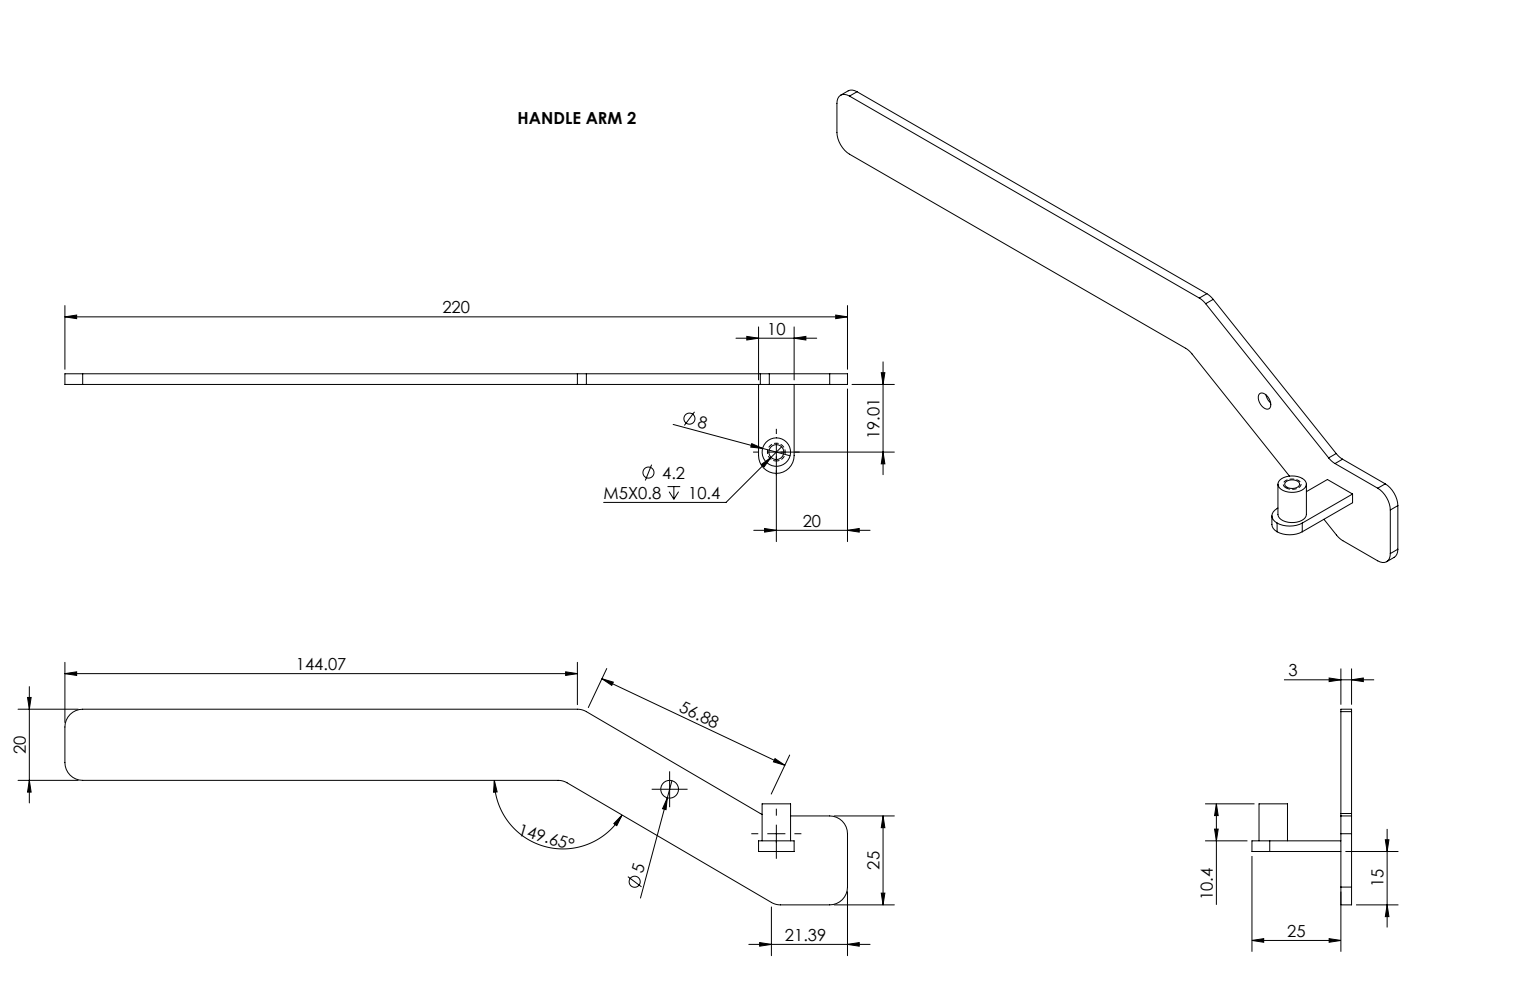
ISO-10303-21;
HEADER;
FILE_DESCRIPTION (('STEP AP214'),
    '1' );
FILE_NAME ('Handle arm 2.step',
    '2026-09-24T10:15:42',
    ( '' ),
    ( '' ),
    'SwSTEP 2.0',
    'SolidWorks 2026',
    '' );
FILE_SCHEMA (( 'AUTOMOTIVE_DESIGN' ));
ENDSEC;

DATA;
#2=DIRECTION ( 'NONE',  ( 0.000000000000000000, 0.000000000000000000, -1.000000000000000000 ) ) ;
#46=CARTESIAN_POINT ( 'NONE',  ( 3.686287386450715076E-15, -27.00000000000000000, 25.01316734529526187 ) ) ;
#85=EDGE_CURVE ( 'NONE', #9356, #911, #14003, .T. ) ;
#87=DIRECTION ( 'NONE',  ( 0.000000000000000000, 0.000000000000000000, 1.000000000000000000 ) ) ;
#167=AXIS2_PLACEMENT_3D ( 'NONE', #17284, #15857, #10023 ) ;
#171=CARTESIAN_POINT ( 'NONE',  ( 3.686287386450715076E-15, -16.60000000000000142, 27.11316734529526329 ) ) ;
#182=VERTEX_POINT ( 'NONE', #619 ) ;
#190=VECTOR ( 'NONE', #11538, 1000.000000000000000 ) ;
#196=DIRECTION ( 'NONE',  ( -0.000000000000000000, 1.000000000000000000, -0.000000000000000000 ) ) ;
#211=AXIS2_PLACEMENT_3D ( 'NONE', #14150, #17206, #1054 ) ;
#237=FACE_OUTER_BOUND ( 'NONE', #12508, .T. ) ;
#244=( LENGTH_UNIT ( ) NAMED_UNIT ( * ) SI_UNIT ( .MILLI., .METRE. ) );
#245=DIRECTION ( 'NONE',  ( 0.000000000000000000, 0.000000000000000000, 1.000000000000000000 ) ) ;
#255=ORIENTED_EDGE ( 'NONE', *, *, #85, .F. ) ;
#262=ORIENTED_EDGE ( 'NONE', *, *, #15287, .T. ) ;
#268=ADVANCED_FACE ( 'NONE', ( #16665 ), #15218, .F. ) ;
#282=EDGE_LOOP ( 'NONE', ( #350, #8843, #5301, #9575 ) ) ;
#335=CARTESIAN_POINT ( 'NONE',  ( -54.57590088527786065, 9.999999999999973355, 6.000000000000000000 ) ) ;
#350=ORIENTED_EDGE ( 'NONE', *, *, #847, .F. ) ;
#355=DIRECTION ( 'NONE',  ( -0.000000000000000000, 1.000000000000000000, -0.000000000000000000 ) ) ;
#372=DIRECTION ( 'NONE',  ( 0.000000000000000000, 0.000000000000000000, 1.000000000000000000 ) ) ;
#375=EDGE_CURVE ( 'NONE', #5396, #13349, #1164, .T. ) ;
#384=CARTESIAN_POINT ( 'NONE',  ( 20.00000000000000711, -45.00000000000000000, 6.000000000000000000 ) ) ;
#390=ORIENTED_EDGE ( 'NONE', *, *, #17273, .T. ) ;
#427=SURFACE_SIDE_STYLE ('',( #3278 ) ) ;
#479=PLANE ( 'NONE',  #15685 ) ;
#484=LINE ( 'NONE', #384, #10360 ) ;
#503=( GEOMETRIC_REPRESENTATION_CONTEXT ( 3 ) GLOBAL_UNCERTAINTY_ASSIGNED_CONTEXT ( ( #10335 ) ) GLOBAL_UNIT_ASSIGNED_CONTEXT ( ( #244, #6073, #17536 ) ) REPRESENTATION_CONTEXT ( 'NONE', 'WORKASPACE' ) );
#516=ORIENTED_EDGE ( 'NONE', *, *, #14577, .T. ) ;
#552=ORIENTED_EDGE ( 'NONE', *, *, #12638, .T. ) ;
#553=ORIENTED_EDGE ( 'NONE', *, *, #2654, .T. ) ;
#578=FACE_BOUND ( 'NONE', #591, .T. ) ;
#581=EDGE_CURVE ( 'NONE', #13464, #1391, #8679, .T. ) ;
#591=EDGE_LOOP ( 'NONE', ( #390, #2249 ) ) ;
#619=CARTESIAN_POINT ( 'NONE',  ( 15.00000000000000711, -45.00000000000000000, 6.000000000000000000 ) ) ;
#624=ADVANCED_FACE ( 'NONE', ( #14823 ), #6227, .F. ) ;
#647=CARTESIAN_POINT ( 'NONE',  ( 15.00000000000000711, -19.99999999999999645, 6.000000000000000000 ) ) ;
#656=ORIENTED_EDGE ( 'NONE', *, *, #2270, .T. ) ;
#720=CARTESIAN_POINT ( 'NONE',  ( -61.35602477868047799, -10.00000000000000888, 6.000000000000000000 ) ) ;
#722=EDGE_CURVE ( 'NONE', #14617, #1651, #2384, .T. ) ;
#738=VECTOR ( 'NONE', #4589, 1000.000000000000227 ) ;
#785=CARTESIAN_POINT ( 'NONE',  ( 5.000000000000006217, -30.00000000000000000, 6.000000000000000000 ) ) ;
#789=DIRECTION ( 'NONE',  ( 0.000000000000000000, 0.000000000000000000, -1.000000000000000000 ) ) ;
#825=CIRCLE ( 'NONE', #211, 5.000000000000004441 ) ;
#831=DIRECTION ( 'NONE',  ( 1.000000000000000000, 0.000000000000000000, 0.000000000000000000 ) ) ;
#836=CARTESIAN_POINT ( 'NONE',  ( 15.00000000000000711, -40.00000000000000000, 3.000000000000000000 ) ) ;
#840=ORIENTED_EDGE ( 'NONE', *, *, #14124, .T. ) ;
#846=VERTEX_POINT ( 'NONE', #13076 ) ;
#847=EDGE_CURVE ( 'NONE', #1377, #13406, #12495, .T. ) ;
#858=DIRECTION ( 'NONE',  ( -1.000000000000000000, -0.000000000000000000, -0.000000000000000000 ) ) ;
#904=CARTESIAN_POINT ( 'NONE',  ( 15.00000000000000711, -24.99999999999999645, 6.000000000000000000 ) ) ;
#911=VERTEX_POINT ( 'NONE', #7070 ) ;
#976=ADVANCED_FACE ( 'NONE', ( #6303 ), #14988, .F. ) ;
#983=CARTESIAN_POINT ( 'NONE',  ( -4.999999999999995559, -30.00000000000000000, 26.00000000000000000 ) ) ;
#994=ORIENTED_EDGE ( 'NONE', *, *, #17881, .T. ) ;
#998=VERTEX_POINT ( 'NONE', #13172 ) ;
#1009=AXIS2_PLACEMENT_3D ( 'NONE', #5627, #10227, #11663 ) ;
#1054=DIRECTION ( 'NONE',  ( -1.000000000000000000, 0.000000000000000000, 0.000000000000000000 ) ) ;
#1056=DIRECTION ( 'NONE',  ( 0.000000000000000000, 0.000000000000000000, -1.000000000000000000 ) ) ;
#1088=AXIS2_PLACEMENT_3D ( 'NONE', #17339, #4255, #4345 ) ;
#1150=LINE ( 'NONE', #9834, #4116 ) ;
#1156=FACE_OUTER_BOUND ( 'NONE', #9724, .T. ) ;
#1164=CIRCLE ( 'NONE', #7602, 5.000000000000004441 ) ;
#1180=DIRECTION ( 'NONE',  ( 0.000000000000000000, 0.000000000000000000, 1.000000000000000000 ) ) ;
#1181=DIRECTION ( 'NONE',  ( -0.000000000000000000, -0.000000000000000000, -1.000000000000000000 ) ) ;
#1190=ORIENTED_EDGE ( 'NONE', *, *, #7855, .T. ) ;
#1216=CARTESIAN_POINT ( 'NONE',  ( -4.505465888036630062, -19.31487138727242581, 6.000000000000000000 ) ) ;
#1227=DIRECTION ( 'NONE',  ( 0.000000000000000000, 0.000000000000000000, -1.000000000000000000 ) ) ;
#1238=DIRECTION ( 'NONE',  ( -0.000000000000000000, -0.000000000000000000, 1.000000000000000000 ) ) ;
#1254=CARTESIAN_POINT ( 'NONE',  ( 20.00000000000000711, -24.99999999999999645, 6.000000000000000000 ) ) ;
#1255=FACE_OUTER_BOUND ( 'NONE', #3235, .T. ) ;
#1285=EDGE_CURVE ( 'NONE', #10015, #2548, #5780, .T. ) ;
#1289=LINE ( 'NONE', #9710, #13681 ) ;
#1297=ORIENTED_EDGE ( 'NONE', *, *, #5077, .T. ) ;
#1326=CARTESIAN_POINT ( 'NONE',  ( -54.57590088527786065, 9.999999999999973355, 6.000000000000000000 ) ) ;
#1336=FACE_OUTER_BOUND ( 'NONE', #12011, .T. ) ;
#1377=VERTEX_POINT ( 'NONE', #7431 ) ;
#1391=VERTEX_POINT ( 'NONE', #12012 ) ;
#1419=CARTESIAN_POINT ( 'NONE',  ( 4.336808689942014581E-15, -27.00000000000000000, 26.00000000000000000 ) ) ;
#1431=AXIS2_PLACEMENT_3D ( 'NONE', #13888, #9216, #7903 ) ;
#1441=FACE_OUTER_BOUND ( 'NONE', #12105, .T. ) ;
#1454=DIRECTION ( 'NONE',  ( -0.000000000000000000, -0.000000000000000000, -1.000000000000000000 ) ) ;
#1517=ORIENTED_EDGE ( 'NONE', *, *, #11103, .F. ) ;
#1518=VERTEX_POINT ( 'NONE', #13981 ) ;
#1519=ORIENTED_EDGE ( 'NONE', *, *, #5489, .T. ) ;
#1529=DIRECTION ( 'NONE',  ( -0.000000000000000000, 1.000000000000000000, -0.000000000000000000 ) ) ;
#1546=DIRECTION ( 'NONE',  ( -0.000000000000000000, -0.000000000000000000, 1.000000000000000000 ) ) ;
#1578=LINE ( 'NONE', #7419, #10628 ) ;
#1586=EDGE_CURVE ( 'NONE', #1391, #14370, #11676, .T. ) ;
#1590=ORIENTED_EDGE ( 'NONE', *, *, #9778, .T. ) ;
#1591=LINE ( 'NONE', #7435, #8998 ) ;
#1605=EDGE_LOOP ( 'NONE', ( #14578, #7944, #5603, #3741, #6106 ) ) ;
#1651=VERTEX_POINT ( 'NONE', #10339 ) ;
#1708=DIRECTION ( 'NONE',  ( 0.000000000000000000, -1.000000000000000000, 0.000000000000000000 ) ) ;
#1717=PLANE ( 'NONE',  #10053 ) ;
#1735=DIRECTION ( 'NONE',  ( -0.8629742774544859607, 0.5052478564545405115, 0.000000000000000000 ) ) ;
#1738=ORIENTED_EDGE ( 'NONE', *, *, #18088, .F. ) ;
#1764=FILL_AREA_STYLE ('',( #3572 ) ) ;
#1774=DIRECTION ( 'NONE',  ( -0.000000000000000000, -0.000000000000000000, 1.000000000000000000 ) ) ;
#1809=DIRECTION ( 'NONE',  ( 0.000000000000000000, 1.000000000000000000, -0.000000000000000000 ) ) ;
#1813=CARTESIAN_POINT ( 'NONE',  ( -53.40568638168567617, 9.314871387272408043, 6.000000000000000000 ) ) ;
#1816=EDGE_CURVE ( 'NONE', #15520, #5678, #15774, .T. ) ;
#1868=DIRECTION ( 'NONE',  ( -1.000000000000000000, -1.387778780781445676E-15, 0.000000000000000000 ) ) ;
#1869=ADVANCED_FACE ( 'NONE', ( #12519 ), #10124, .F. ) ;
#1871=CARTESIAN_POINT ( 'NONE',  ( -58.82978549640777288, -10.68512861272757952, 6.000000000000000000 ) ) ;
#1882=EDGE_LOOP ( 'NONE', ( #10890, #7353 ) ) ;
#1890=ADVANCED_FACE ( 'NONE', ( #10319 ), #15948, .T. ) ;
#1897=DIRECTION ( 'NONE',  ( 0.000000000000000000, -1.000000000000000000, 0.000000000000000000 ) ) ;
#1903=ORIENTED_EDGE ( 'NONE', *, *, #8948, .T. ) ;
#1915=CARTESIAN_POINT ( 'NONE',  ( 3.686287386450715076E-15, -16.60000000000000142, 27.11316734529526329 ) ) ;
#1919=EDGE_CURVE ( 'NONE', #7625, #1518, #14240, .T. ) ;
#1942=EDGE_LOOP ( 'NONE', ( #12597, #3775, #16274, #14695 ) ) ;
#1963=PLANE ( 'NONE',  #5380 ) ;
#1978=ORIENTED_EDGE ( 'NONE', *, *, #8575, .T. ) ;
#1985=DIRECTION ( 'NONE',  ( 1.000000000000000000, 0.000000000000000000, 0.000000000000000000 ) ) ;
#2030=AXIS2_PLACEMENT_3D ( 'NONE', #15716, #11248, #17249 ) ;
#2054=VECTOR ( 'NONE', #11619, 1000.000000000000000 ) ;
#2059=DIRECTION ( 'NONE',  ( 0.000000000000000000, 0.000000000000000000, -1.000000000000000000 ) ) ;
#2077=EDGE_LOOP ( 'NONE', ( #13785, #14387, #12473, #3682 ) ) ;
#2078=ORIENTED_EDGE ( 'NONE', *, *, #17877, .T. ) ;
#2199=LINE ( 'NONE', #16475, #8487 ) ;
#2216=LINE ( 'NONE', #785, #17824 ) ;
#2244=EDGE_CURVE ( 'NONE', #18846, #1377, #4850, .T. ) ;
#2249=ORIENTED_EDGE ( 'NONE', *, *, #2491, .T. ) ;
#2262=DIRECTION ( 'NONE',  ( -0.000000000000000000, -0.000000000000000000, -1.000000000000000000 ) ) ;
#2270=EDGE_CURVE ( 'NONE', #9430, #14370, #1591, .T. ) ;
#2274=ORIENTED_EDGE ( 'NONE', *, *, #18088, .T. ) ;
#2280=CARTESIAN_POINT ( 'NONE',  ( -55.93192566395838128, 9.999999999999973355, 6.000000000000000000 ) ) ;
#2298=CYLINDRICAL_SURFACE ( 'NONE', #3949, 2.499999999999992006 ) ;
#2316=VERTEX_POINT ( 'NONE', #16125 ) ;
#2335=CARTESIAN_POINT ( 'NONE',  ( -30.00000000000000355, -12.50000000000000178, 3.000000000000000000 ) ) ;
#2356=DIRECTION ( 'NONE',  ( -1.000000000000000000, 0.000000000000000000, 0.000000000000000000 ) ) ;
#2371=AXIS2_PLACEMENT_3D ( 'NONE', #17344, #17739, #11904 ) ;
#2382=EDGE_CURVE ( 'NONE', #13257, #7625, #18395, .T. ) ;
#2384=LINE ( 'NONE', #15566, #10687 ) ;
#2394=CARTESIAN_POINT ( 'NONE',  ( -61.35602477868047799, -15.00000000000000711, 6.000000000000000000 ) ) ;
#2491=EDGE_CURVE ( 'NONE', #2548, #14769, #13939, .T. ) ;
#2504=DIRECTION ( 'NONE',  ( -1.000000000000000000, 0.000000000000000000, 0.000000000000000000 ) ) ;
#2511=ORIENTED_EDGE ( 'NONE', *, *, #3757, .T. ) ;
#2528=EDGE_CURVE ( 'NONE', #7625, #15007, #18216, .T. ) ;
#2541=PRODUCT_DEFINITION_FORMATION_WITH_SPECIFIED_SOURCE ( 'ANY', '', #12278, .NOT_KNOWN. ) ;
#2548=VERTEX_POINT ( 'NONE', #5961 ) ;
#2566=EDGE_CURVE ( 'NONE', #18408, #6600, #3875, .T. ) ;
#2588=DIRECTION ( 'NONE',  ( 1.000000000000000000, -0.000000000000000000, -0.000000000000000000 ) ) ;
#2595=CARTESIAN_POINT ( 'NONE',  ( -59.99999999999997158, -10.00000000000000888, 6.000000000000000000 ) ) ;
#2605=ORIENTED_EDGE ( 'NONE', *, *, #2244, .T. ) ;
#2647=AXIS2_PLACEMENT_3D ( 'NONE', #6461, #6559, #18480 ) ;
#2649=ORIENTED_EDGE ( 'NONE', *, *, #9078, .F. ) ;
#2652=ORIENTED_EDGE ( 'NONE', *, *, #14147, .F. ) ;
#2654=EDGE_CURVE ( 'NONE', #15726, #12603, #6937, .T. ) ;
#2689=CARTESIAN_POINT ( 'NONE',  ( -30.00000000000000355, -12.50000000000000178, 6.000000000000000000 ) ) ;
#2695=EDGE_CURVE ( 'NONE', #9382, #15782, #9499, .T. ) ;
#2709=( NAMED_UNIT ( * ) SI_UNIT ( $, .STERADIAN. ) SOLID_ANGLE_UNIT ( ) );
#2724=ORIENTED_EDGE ( 'NONE', *, *, #4872, .F. ) ;
#2744=LINE ( 'NONE', #1326, #5606 ) ;
#2770=DIRECTION ( 'NONE',  ( -1.000000000000000000, 0.000000000000000000, 0.000000000000000000 ) ) ;
#2803=VERTEX_POINT ( 'NONE', #983 ) ;
#2805=VERTEX_POINT ( 'NONE', #8433 ) ;
#2830=VECTOR ( 'NONE', #196, 1000.000000000000000 ) ;
#2892=AXIS2_PLACEMENT_3D ( 'NONE', #15262, #831, #14097 ) ;
#2895=CARTESIAN_POINT ( 'NONE',  ( -53.40568638168567617, 9.314871387272408043, 3.000000000000000000 ) ) ;
#2902=AXIS2_PLACEMENT_3D ( 'NONE', #12160, #10430, #8893 ) ;
#2918=VECTOR ( 'NONE', #16196, 1000.000000000000000 ) ;
#2931=ORIENTED_EDGE ( 'NONE', *, *, #722, .T. ) ;
#2939=AXIS2_PLACEMENT_3D ( 'NONE', #7030, #12844, #11425 ) ;
#2988=CARTESIAN_POINT ( 'NONE',  ( 3.686287386450715076E-15, -27.00000000000000000, 25.01316734529526187 ) ) ;
#2990=DIRECTION ( 'NONE',  ( 0.000000000000000000, 0.000000000000000000, -1.000000000000000000 ) ) ;
#3016=AXIS2_PLACEMENT_3D ( 'NONE', #6543, #17924, #13612 ) ;
#3048=CARTESIAN_POINT ( 'NONE',  ( -0.2192422490275049152, -45.00000000000000000, 6.000000000000000000 ) ) ;
#3049=UNCERTAINTY_MEASURE_WITH_UNIT (LENGTH_MEASURE( 1.000000000000000082E-05 ), #15530, 'distance_accuracy_value', 'NONE');
#3053=CARTESIAN_POINT ( 'NONE',  ( 15.00000000000000711, -24.99999999999999645, 6.000000000000000000 ) ) ;
#3055=CARTESIAN_POINT ( 'NONE',  ( 20.00000000000000711, -40.00000000000000000, 6.000000000000000000 ) ) ;
#3089=PRODUCT_DEFINITION ( 'UNKNOWN', '', #2541, #4217 ) ;
#3113=ORIENTED_EDGE ( 'NONE', *, *, #14292, .T. ) ;
#3126=CARTESIAN_POINT ( 'NONE',  ( -4.999999999999995559, -27.00000000000000000, 31.00000000000000000 ) ) ;
#3143=VECTOR ( 'NONE', #17164, 1000.000000000000000 ) ;
#3145=VERTEX_POINT ( 'NONE', #14221 ) ;
#3169=VERTEX_POINT ( 'NONE', #9908 ) ;
#3179=LINE ( 'NONE', #4545, #8102 ) ;
#3182=CARTESIAN_POINT ( 'NONE',  ( -194.9999999999999716, -5.000000000000024869, 3.000000000000000000 ) ) ;
#3187=AXIS2_PLACEMENT_3D ( 'NONE', #18811, #1708, #7167 ) ;
#3225=DIRECTION ( 'NONE',  ( 0.000000000000000000, -1.000000000000000000, 0.000000000000000000 ) ) ;
#3235=EDGE_LOOP ( 'NONE', ( #3338, #5545, #6726, #16756 ) ) ;
#3246=ORIENTED_EDGE ( 'NONE', *, *, #2566, .T. ) ;
#3251=ORIENTED_EDGE ( 'NONE', *, *, #8948, .F. ) ;
#3258=CIRCLE ( 'NONE', #13950, 5.000000000000000888 ) ;
#3260=ORIENTED_EDGE ( 'NONE', *, *, #13945, .T. ) ;
#3265=FACE_OUTER_BOUND ( 'NONE', #14790, .T. ) ;
#3271=EDGE_CURVE ( 'NONE', #12603, #4207, #17956, .T. ) ;
#3278=SURFACE_STYLE_FILL_AREA ( #1764 ) ;
#3283=FILL_AREA_STYLE ('',( #14663 ) ) ;
#3291=EDGE_LOOP ( 'NONE', ( #11241, #8275, #18451, #8539 ) ) ;
#3310=CARTESIAN_POINT ( 'NONE',  ( 3.686287386450715076E-15, -16.60000000000000142, 25.01316734529526187 ) ) ;
#3338=ORIENTED_EDGE ( 'NONE', *, *, #15287, .F. ) ;
#3364=DIRECTION ( 'NONE',  ( -1.000000000000000000, 0.000000000000000000, 0.000000000000000000 ) ) ;
#3379=CARTESIAN_POINT ( 'NONE',  ( 4.336808689942017736E-15, 0.000000000000000000, 31.00000000000000000 ) ) ;
#3402=VECTOR ( 'NONE', #3460, 1000.000000000000000 ) ;
#3414=AXIS2_PLACEMENT_3D ( 'NONE', #16438, #372, #16716 ) ;
#3444=CIRCLE ( 'NONE', #7737, 5.000000000000004441 ) ;
#3445=ORIENTED_EDGE ( 'NONE', *, *, #11834, .F. ) ;
#3457=LINE ( 'NONE', #13493, #16294 ) ;
#3460=DIRECTION ( 'NONE',  ( -0.8629742774544855166, 0.5052478564545411777, -0.000000000000000000 ) ) ;
#3480=DIRECTION ( 'NONE',  ( 5.782411586589358625E-16, -1.000000000000000000, -0.000000000000000000 ) ) ;
#3493=ORIENTED_EDGE ( 'NONE', *, *, #11591, .F. ) ;
#3521=ADVANCED_FACE ( 'NONE', ( #237 ), #11349, .T. ) ;
#3553=MANIFOLD_SOLID_BREP ( 'AdvancedHole1', #9975 ) ;
#3563=VERTEX_POINT ( 'NONE', #6162 ) ;
#3565=DIRECTION ( 'NONE',  ( 0.000000000000000000, 0.000000000000000000, 1.000000000000000000 ) ) ;
#3572=FILL_AREA_STYLE_COLOUR ( '', #16481 ) ;
#3603=EDGE_CURVE ( 'NONE', #10015, #2805, #7629, .T. ) ;
#3604=PLANE ( 'NONE',  #2892 ) ;
#3671=PRODUCT_CONTEXT ( 'NONE', #11932, 'mechanical' ) ;
#3675=CIRCLE ( 'NONE', #4289, 4.000000000000000000 ) ;
#3682=ORIENTED_EDGE ( 'NONE', *, *, #16814, .F. ) ;
#3695=ADVANCED_FACE ( 'NONE', ( #6642 ), #7005, .T. ) ;
#3696=LINE ( 'NONE', #15350, #10169 ) ;
#3741=ORIENTED_EDGE ( 'NONE', *, *, #4041, .T. ) ;
#3755=ADVANCED_FACE ( 'NONE', ( #1255 ), #15970, .T. ) ;
#3757=EDGE_CURVE ( 'NONE', #2803, #14617, #12914, .T. ) ;
#3775=ORIENTED_EDGE ( 'NONE', *, *, #18129, .T. ) ;
#3782=FACE_OUTER_BOUND ( 'NONE', #6562, .T. ) ;
#3815=AXIS2_PLACEMENT_3D ( 'NONE', #4441, #8744, #14567 ) ;
#3817=EDGE_LOOP ( 'NONE', ( #9700, #10501, #8493, #2511, #2931 ) ) ;
#3828=CARTESIAN_POINT ( 'NONE',  ( -4.999999999999995559, -27.00000000000000000, 6.000000000000000000 ) ) ;
#3841=AXIS2_PLACEMENT_3D ( 'NONE', #17972, #12233, #16622 ) ;
#3875=CIRCLE ( 'NONE', #9061, 5.000000000000000000 ) ;
#3881=AXIS2_PLACEMENT_3D ( 'NONE', #8923, #13711, #7705 ) ;
#3898=CARTESIAN_POINT ( 'NONE',  ( 5.000000000000004441, -27.00000000000000000, 31.00000000000000000 ) ) ;
#3906=CIRCLE ( 'NONE', #17034, 5.000000000000000000 ) ;
#3912=FACE_OUTER_BOUND ( 'NONE', #7626, .T. ) ;
#3915=ADVANCED_FACE ( 'NONE', ( #18266 ), #2298, .F. ) ;
#3935=CARTESIAN_POINT ( 'NONE',  ( -199.9999999999999716, -10.00000000000002665, 6.000000000000000000 ) ) ;
#3949=AXIS2_PLACEMENT_3D ( 'NONE', #5355, #15392, #10924 ) ;
#3958=DIRECTION ( 'NONE',  ( 1.000000000000000000, 0.000000000000000000, 0.000000000000000000 ) ) ;
#3959=DIRECTION ( 'NONE',  ( -0.000000000000000000, -1.000000000000000000, -0.000000000000000000 ) ) ;
#3962=VERTEX_POINT ( 'NONE', #3828 ) ;
#3980=ORIENTED_EDGE ( 'NONE', *, *, #8436, .F. ) ;
#3986=ORIENTED_EDGE ( 'NONE', *, *, #15577, .T. ) ;
#3995=FACE_OUTER_BOUND ( 'NONE', #9987, .T. ) ;
#4022=CARTESIAN_POINT ( 'NONE',  ( -199.9999999999999716, -5.000000000000024869, 6.000000000000000000 ) ) ;
#4041=EDGE_CURVE ( 'NONE', #3145, #3962, #14334, .T. ) ;
#4059=CIRCLE ( 'NONE', #11680, 4.000000000000000000 ) ;
#4113=AXIS2_PLACEMENT_3D ( 'NONE', #17385, #10217, #11564 ) ;
#4116=VECTOR ( 'NONE', #16051, 1000.000000000000227 ) ;
#4135=EDGE_CURVE ( 'NONE', #12673, #911, #18818, .T. ) ;
#4158=MECHANICAL_DESIGN_GEOMETRIC_PRESENTATION_REPRESENTATION('',(#6598),#503);
#4175=ORIENTED_EDGE ( 'NONE', *, *, #4872, .T. ) ;
#4207=VERTEX_POINT ( 'NONE', #1915 ) ;
#4211=CARTESIAN_POINT ( 'NONE',  ( 3.686287386450715076E-15, -27.00000000000000000, 25.01316734529526187 ) ) ;
#4217=PRODUCT_DEFINITION_CONTEXT ( 'detailed design', #14375, 'design' ) ;
#4255=DIRECTION ( 'NONE',  ( -0.000000000000000000, -0.000000000000000000, 1.000000000000000000 ) ) ;
#4264=AXIS2_PLACEMENT_3D ( 'NONE', #8501, #1227, #7165 ) ;
#4272=CARTESIAN_POINT ( 'NONE',  ( 4.176146106109656457E-15, -16.60000000000000142, 29.01316734529526187 ) ) ;
#4289=AXIS2_PLACEMENT_3D ( 'NONE', #4211, #5813, #9832 ) ;
#4306=LINE ( 'NONE', #5817, #2830 ) ;
#4322=DIRECTION ( 'NONE',  ( -1.000000000000000000, 0.000000000000000000, 0.000000000000000000 ) ) ;
#4345=DIRECTION ( 'NONE',  ( -1.000000000000000000, 0.000000000000000000, 0.000000000000000000 ) ) ;
#4350=SURFACE_STYLE_FILL_AREA ( #3283 ) ;
#4377=ORIENTED_EDGE ( 'NONE', *, *, #5439, .T. ) ;
#4384=AXIS2_PLACEMENT_3D ( 'NONE', #9240, #4564, #1985 ) ;
#4408=AXIS2_PLACEMENT_3D ( 'NONE', #12984, #11657, #8506 ) ;
#4413=EDGE_CURVE ( 'NONE', #3962, #14617, #15736, .T. ) ;
#4431=ORIENTED_EDGE ( 'NONE', *, *, #16809, .T. ) ;
#4441=CARTESIAN_POINT ( 'NONE',  ( -4.999999999999995559, -30.00000000000000000, 31.00000000000000000 ) ) ;
#4444=PRESENTATION_STYLE_ASSIGNMENT (( #7417 ) ) ;
#4453=ORIENTED_EDGE ( 'NONE', *, *, #2566, .F. ) ;
#4454=EDGE_LOOP ( 'NONE', ( #8547, #16780, #7578 ) ) ;
#4456=CIRCLE ( 'NONE', #1088, 5.000000000000004441 ) ;
#4498=CARTESIAN_POINT ( 'NONE',  ( -199.9999999999999716, -10.00000000000002665, 6.000000000000000000 ) ) ;
#4545=CARTESIAN_POINT ( 'NONE',  ( -59.99999999999997158, -10.00000000000000888, 3.000000000000000000 ) ) ;
#4548=FACE_OUTER_BOUND ( 'NONE', #7524, .T. ) ;
#4561=DIRECTION ( 'NONE',  ( -1.000000000000000000, -5.782411586589358625E-16, 0.000000000000000000 ) ) ;
#4564=DIRECTION ( 'NONE',  ( 0.000000000000000000, 0.000000000000000000, 1.000000000000000000 ) ) ;
#4570=DIRECTION ( 'NONE',  ( 0.000000000000000000, 0.000000000000000000, -1.000000000000000000 ) ) ;
#4577=ORIENTED_EDGE ( 'NONE', *, *, #12513, .T. ) ;
#4584=CARTESIAN_POINT ( 'NONE',  ( -55.93192566395838128, 9.999999999999973355, 3.000000000000000000 ) ) ;
#4589=DIRECTION ( 'NONE',  ( 0.8629742774544859607, -0.5052478564545405115, -0.000000000000000000 ) ) ;
#4590=DIRECTION ( 'NONE',  ( 1.000000000000000000, 0.000000000000000000, 0.000000000000000000 ) ) ;
#4627=CARTESIAN_POINT ( 'NONE',  ( 3.686287386450715076E-15, -27.00000000000000000, 25.01316734529526187 ) ) ;
#4643=CARTESIAN_POINT ( 'NONE',  ( -199.9999999999999716, -5.000000000000024869, 6.000000000000000000 ) ) ;
#4644=EDGE_CURVE ( 'NONE', #14303, #15038, #13554, .T. ) ;
#4648=ORIENTED_EDGE ( 'NONE', *, *, #2382, .F. ) ;
#4684=DIRECTION ( 'NONE',  ( 0.000000000000000000, 0.000000000000000000, 1.000000000000000000 ) ) ;
#4706=DIRECTION ( 'NONE',  ( 1.049727191138619928E-16, 0.5150380749100523792, -0.8571673007021134438 ) ) ;
#4736=DIRECTION ( 'NONE',  ( -1.000000000000000000, 0.000000000000000000, 0.000000000000000000 ) ) ;
#4758=DIRECTION ( 'NONE',  ( -0.000000000000000000, 1.000000000000000000, -0.000000000000000000 ) ) ;
#4769=EDGE_CURVE ( 'NONE', #846, #3169, #11560, .T. ) ;
#4789=LINE ( 'NONE', #12247, #16996 ) ;
#4840=LINE ( 'NONE', #720, #11810 ) ;
#4850=LINE ( 'NONE', #7633, #18753 ) ;
#4872=EDGE_CURVE ( 'NONE', #13406, #8344, #2744, .T. ) ;
#4882=( GEOMETRIC_REPRESENTATION_CONTEXT ( 3 ) GLOBAL_UNCERTAINTY_ASSIGNED_CONTEXT ( ( #11314 ) ) GLOBAL_UNIT_ASSIGNED_CONTEXT ( ( #10749, #6361, #15236 ) ) REPRESENTATION_CONTEXT ( 'NONE', 'WORKASPACE' ) );
#4920=PRESENTATION_STYLE_ASSIGNMENT (( #15043 ) ) ;
#4929=CARTESIAN_POINT ( 'NONE',  ( -27.50000000000000711, -12.50000000000000178, 3.000000000000000000 ) ) ;
#4957=ADVANCED_FACE ( 'NONE', ( #7748, #13370 ), #479, .F. ) ;
#4963=PLANE ( 'NONE',  #5345 ) ;
#4992=ORIENTED_EDGE ( 'NONE', *, *, #1919, .T. ) ;
#5010=ADVANCED_FACE ( 'NONE', ( #5475 ), #5744, .F. ) ;
#5077=EDGE_CURVE ( 'NONE', #18014, #2316, #16619, .T. ) ;
#5082=CARTESIAN_POINT ( 'NONE',  ( -54.57590088527786065, 9.999999999999973355, 3.000000000000000000 ) ) ;
#5098=VECTOR ( 'NONE', #1181, 1000.000000000000000 ) ;
#5106=VECTOR ( 'NONE', #1546, 1000.000000000000000 ) ;
#5115=CARTESIAN_POINT ( 'NONE',  ( 3.943463214271659518E-15, -16.60000000000000142, 22.91316734529526045 ) ) ;
#5130=CARTESIAN_POINT ( 'NONE',  ( 15.00000000000000711, -40.00000000000000000, 6.000000000000000000 ) ) ;
#5145=LINE ( 'NONE', #3898, #14518 ) ;
#5176=CARTESIAN_POINT ( 'NONE',  ( 15.00000000000000711, -19.99999999999999645, 6.000000000000000000 ) ) ;
#5212=ORIENTED_EDGE ( 'NONE', *, *, #14729, .T. ) ;
#5225=CARTESIAN_POINT ( 'NONE',  ( -1.389456752619696367, -44.31487138727242581, 6.000000000000000000 ) ) ;
#5301=ORIENTED_EDGE ( 'NONE', *, *, #14124, .F. ) ;
#5319=VECTOR ( 'NONE', #16971, 1000.000000000000000 ) ;
#5327=ORIENTED_EDGE ( 'NONE', *, *, #17881, .F. ) ;
#5335=PLANE ( 'NONE',  #7776 ) ;
#5345=AXIS2_PLACEMENT_3D ( 'NONE', #3126, #3225, #7943 ) ;
#5347=EDGE_CURVE ( 'NONE', #3169, #1518, #825, .T. ) ;
#5355=CARTESIAN_POINT ( 'NONE',  ( -30.00000000000000355, -12.50000000000000178, 6.000000000000000000 ) ) ;
#5360=CARTESIAN_POINT ( 'NONE',  ( -32.49999999999999289, -12.50000000000000178, 6.000000000000000000 ) ) ;
#5380=AXIS2_PLACEMENT_3D ( 'NONE', #335, #13226, #6163 ) ;
#5396=VERTEX_POINT ( 'NONE', #4022 ) ;
#5398=ORIENTED_EDGE ( 'NONE', *, *, #4135, .T. ) ;
#5406=DIRECTION ( 'NONE',  ( 0.000000000000000000, 0.000000000000000000, -1.000000000000000000 ) ) ;
#5439=EDGE_CURVE ( 'NONE', #5705, #10186, #7549, .T. ) ;
#5462=DIRECTION ( 'NONE',  ( 0.000000000000000000, -1.000000000000000000, 0.000000000000000000 ) ) ;
#5463=CIRCLE ( 'NONE', #6402, 2.100000000000000977 ) ;
#5475=FACE_OUTER_BOUND ( 'NONE', #13295, .T. ) ;
#5478=ORIENTED_EDGE ( 'NONE', *, *, #1586, .T. ) ;
#5481=ORIENTED_EDGE ( 'NONE', *, *, #13945, .F. ) ;
#5489=EDGE_CURVE ( 'NONE', #12673, #16909, #6319, .T. ) ;
#5535=CARTESIAN_POINT ( 'NONE',  ( 3.686287386450715076E-15, -27.00000000000000000, 27.11316734529526329 ) ) ;
#5541=EDGE_LOOP ( 'NONE', ( #1297, #12434, #16868, #17434 ) ) ;
#5545=ORIENTED_EDGE ( 'NONE', *, *, #1586, .F. ) ;
#5556=CARTESIAN_POINT ( 'NONE',  ( -30.00000000000000355, -12.50000000000000178, 6.000000000000000000 ) ) ;
#5600=CARTESIAN_POINT ( 'NONE',  ( -194.9999999999999716, -10.00000000000002665, 6.000000000000000000 ) ) ;
#5603=ORIENTED_EDGE ( 'NONE', *, *, #8436, .T. ) ;
#5606=VECTOR ( 'NONE', #18812, 1000.000000000000000 ) ;
#5627=CARTESIAN_POINT ( 'NONE',  ( 3.686287386450715076E-15, -16.60000000000000142, 25.01316734529526187 ) ) ;
#5647=CONICAL_SURFACE ( 'NONE', #12674, 2.100000000000000977, 1.029744258676656532 ) ;
#5661=ORIENTED_EDGE ( 'NONE', *, *, #9078, .T. ) ;
#5678=VERTEX_POINT ( 'NONE', #15290 ) ;
#5705=VERTEX_POINT ( 'NONE', #17546 ) ;
#5724=ADVANCED_FACE ( 'NONE', ( #8495 ), #14322, .T. ) ;
#5731=ORIENTED_EDGE ( 'NONE', *, *, #14910, .F. ) ;
#5734=ADVANCED_FACE ( 'NONE', ( #3912 ), #15471, .F. ) ;
#5744=CYLINDRICAL_SURFACE ( 'NONE', #9288, 4.999999999999997335 ) ;
#5759=VECTOR ( 'NONE', #14419, 1000.000000000000000 ) ;
#5780=LINE ( 'NONE', #4272, #3143 ) ;
#5797=SHAPE_REPRESENTATION ( 'Handle arm 2', ( #2030 ), #14825 ) ;
#5813=DIRECTION ( 'NONE',  ( 0.000000000000000000, -1.000000000000000000, 0.000000000000000000 ) ) ;
#5817=CARTESIAN_POINT ( 'NONE',  ( 20.00000000000000711, -19.99999999999999645, 3.000000000000000000 ) ) ;
#5822=DIRECTION ( 'NONE',  ( -0.000000000000000000, -0.000000000000000000, 1.000000000000000000 ) ) ;
#5863=PLANE ( 'NONE',  #3815 ) ;
#5870=EDGE_LOOP ( 'NONE', ( #15390, #7937 ) ) ;
#5871=CARTESIAN_POINT ( 'NONE',  ( 3.686287386450715076E-15, -16.60000000000000142, 25.01316734529526187 ) ) ;
#5873=CIRCLE ( 'NONE', #14732, 2.100000000000000977 ) ;
#5890=CYLINDRICAL_SURFACE ( 'NONE', #17248, 4.000000000000000000 ) ;
#5898=VERTEX_POINT ( 'NONE', #5115 ) ;
#5911=FACE_OUTER_BOUND ( 'NONE', #8521, .T. ) ;
#5924=ADVANCED_FACE ( 'NONE', ( #16960 ), #9594, .F. ) ;
#5934=CARTESIAN_POINT ( 'NONE',  ( 3.943463214271659518E-15, -27.00000000000000000, 22.91316734529526045 ) ) ;
#5957=DIRECTION ( 'NONE',  ( 0.000000000000000000, 0.000000000000000000, -1.000000000000000000 ) ) ;
#5961=CARTESIAN_POINT ( 'NONE',  ( 4.176146106109656457E-15, -27.00000000000000000, 29.01316734529526187 ) ) ;
#6028=DIRECTION ( 'NONE',  ( -1.000000000000000000, 0.000000000000000000, 0.000000000000000000 ) ) ;
#6062=ORIENTED_EDGE ( 'NONE', *, *, #14577, .F. ) ;
#6073=( NAMED_UNIT ( * ) PLANE_ANGLE_UNIT ( ) SI_UNIT ( $, .RADIAN. ) );
#6080=VECTOR ( 'NONE', #5462, 1000.000000000000000 ) ;
#6106=ORIENTED_EDGE ( 'NONE', *, *, #15840, .F. ) ;
#6114=DIRECTION ( 'NONE',  ( 0.000000000000000000, -1.000000000000000000, 0.000000000000000000 ) ) ;
#6162=CARTESIAN_POINT ( 'NONE',  ( 4.336808689942017736E-15, -30.00000000000000000, 31.00000000000000000 ) ) ;
#6163=DIRECTION ( 'NONE',  ( 0.8629742774544855166, -0.5052478564545411777, 0.000000000000000000 ) ) ;
#6166=CARTESIAN_POINT ( 'NONE',  ( -58.82978549640777288, -10.68512861272758308, 3.000000000000000000 ) ) ;
#6168=DIRECTION ( 'NONE',  ( -1.000000000000000000, 0.000000000000000000, 0.000000000000000000 ) ) ;
#6171=LINE ( 'NONE', #4643, #2054 ) ;
#6227=PLANE ( 'NONE',  #18489 ) ;
#6243=ORIENTED_EDGE ( 'NONE', *, *, #15577, .F. ) ;
#6303=FACE_OUTER_BOUND ( 'NONE', #7291, .T. ) ;
#6318=ORIENTED_EDGE ( 'NONE', *, *, #7855, .F. ) ;
#6319=CIRCLE ( 'NONE', #16987, 5.000000000000004441 ) ;
#6323=DIRECTION ( 'NONE',  ( -0.000000000000000000, -0.000000000000000000, -1.000000000000000000 ) ) ;
#6324=VECTOR ( 'NONE', #15842, 1000.000000000000000 ) ;
#6331=PRODUCT_DEFINITION_SHAPE ( 'NONE', 'NONE',  #3089 ) ;
#6337=LINE ( 'NONE', #5934, #16471 ) ;
#6361=( NAMED_UNIT ( * ) PLANE_ANGLE_UNIT ( ) SI_UNIT ( $, .RADIAN. ) );
#6364=CARTESIAN_POINT ( 'NONE',  ( 5.000000000000006217, -30.00000000000000000, 26.00000000000000000 ) ) ;
#6402=AXIS2_PLACEMENT_3D ( 'NONE', #14613, #1529, #4684 ) ;
#6461=CARTESIAN_POINT ( 'NONE',  ( -59.99999999999997158, -10.00000000000000888, 6.000000000000000000 ) ) ;
#6523=CARTESIAN_POINT ( 'NONE',  ( 3.686287386450715076E-15, -28.26180729995786933, 25.01316734529526187 ) ) ;
#6543=CARTESIAN_POINT ( 'NONE',  ( 3.686287386450715076E-15, -16.60000000000000142, 25.01316734529526187 ) ) ;
#6559=DIRECTION ( 'NONE',  ( -1.239088197126290570E-16, 1.000000000000000000, 0.000000000000000000 ) ) ;
#6562=EDGE_LOOP ( 'NONE', ( #11555, #2649, #18485, #6318 ) ) ;
#6598=STYLED_ITEM ( 'NONE', ( #4444 ), #18114 ) ;
#6600=VERTEX_POINT ( 'NONE', #13480 ) ;
#6608=VECTOR ( 'NONE', #7632, 1000.000000000000000 ) ;
#6619=DIRECTION ( 'NONE',  ( -5.782411586589358625E-16, 1.000000000000000000, 0.000000000000000000 ) ) ;
#6627=CARTESIAN_POINT ( 'NONE',  ( -4.999999999999995559, -27.00000000000000000, 26.00000000000000000 ) ) ;
#6642=FACE_OUTER_BOUND ( 'NONE', #16962, .T. ) ;
#6661=ORIENTED_EDGE ( 'NONE', *, *, #14022, .T. ) ;
#6694=ORIENTED_EDGE ( 'NONE', *, *, #16781, .T. ) ;
#6725=ORIENTED_EDGE ( 'NONE', *, *, #13748, .F. ) ;
#6726=ORIENTED_EDGE ( 'NONE', *, *, #581, .F. ) ;
#6735=LINE ( 'NONE', #9315, #9013 ) ;
#6744=FACE_OUTER_BOUND ( 'NONE', #11117, .T. ) ;
#6752=ORIENTED_EDGE ( 'NONE', *, *, #16781, .F. ) ;
#6760=DIRECTION ( 'NONE',  ( 0.000000000000000000, -1.000000000000000000, 0.000000000000000000 ) ) ;
#6793=ORIENTED_EDGE ( 'NONE', *, *, #14292, .F. ) ;
#6802=EDGE_CURVE ( 'NONE', #5678, #9382, #14100, .T. ) ;
#6804=DIRECTION ( 'NONE',  ( -1.000000000000000000, 0.000000000000000000, 0.000000000000000000 ) ) ;
#6821=SHAPE_DEFINITION_REPRESENTATION ( #6331, #5797 ) ;
#6833=ORIENTED_EDGE ( 'NONE', *, *, #722, .F. ) ;
#6846=EDGE_CURVE ( 'NONE', #2316, #18014, #10752, .T. ) ;
#6898=DIRECTION ( 'NONE',  ( -1.000000000000000000, 0.000000000000000000, -0.000000000000000000 ) ) ;
#6937=CIRCLE ( 'NONE', #1431, 2.100000000000000977 ) ;
#6951=CARTESIAN_POINT ( 'NONE',  ( -199.9999999999999716, 9.999999999999973355, 6.000000000000000000 ) ) ;
#7000=ORIENTED_EDGE ( 'NONE', *, *, #9289, .T. ) ;
#7005=CYLINDRICAL_SURFACE ( 'NONE', #11892, 4.999999999999997335 ) ;
#7030=CARTESIAN_POINT ( 'NONE',  ( 3.686287386450715076E-15, -27.00000000000000000, 25.01316734529526187 ) ) ;
#7070=CARTESIAN_POINT ( 'NONE',  ( -1.389456752619696367, -44.31487138727242581, 3.000000000000000000 ) ) ;
#7085=DIRECTION ( 'NONE',  ( 0.000000000000000000, 0.000000000000000000, -1.000000000000000000 ) ) ;
#7163=DIRECTION ( 'NONE',  ( -0.000000000000000000, 1.000000000000000000, -0.000000000000000000 ) ) ;
#7165=DIRECTION ( 'NONE',  ( -1.000000000000000000, 0.000000000000000000, 0.000000000000000000 ) ) ;
#7167=DIRECTION ( 'NONE',  ( 0.000000000000000000, -0.000000000000000000, -1.000000000000000000 ) ) ;
#7268=FACE_OUTER_BOUND ( 'NONE', #11369, .T. ) ;
#7291=EDGE_LOOP ( 'NONE', ( #16933, #12009, #4431, #5661 ) ) ;
#7307=ORIENTED_EDGE ( 'NONE', *, *, #2528, .T. ) ;
#7314=VECTOR ( 'NONE', #16851, 1000.000000000000000 ) ;
#7321=LINE ( 'NONE', #6166, #17868 ) ;
#7331=DIRECTION ( 'NONE',  ( 0.000000000000000000, 0.000000000000000000, -1.000000000000000000 ) ) ;
#7353=ORIENTED_EDGE ( 'NONE', *, *, #17360, .F. ) ;
#7417=SURFACE_STYLE_USAGE ( .BOTH. , #11707 ) ;
#7419=CARTESIAN_POINT ( 'NONE',  ( -194.9999999999999716, 9.999999999999973355, 6.000000000000000000 ) ) ;
#7431=CARTESIAN_POINT ( 'NONE',  ( -1.979226605763932723, -19.99999999999999645, 6.000000000000000000 ) ) ;
#7435=CARTESIAN_POINT ( 'NONE',  ( 20.00000000000000711, -19.99999999999999645, 6.000000000000000000 ) ) ;
#7451=ORIENTED_EDGE ( 'NONE', *, *, #375, .F. ) ;
#7469=AXIS2_PLACEMENT_3D ( 'NONE', #5556, #17227, #10156 ) ;
#7480=EDGE_LOOP ( 'NONE', ( #16037, #10474, #17253, #2274 ) ) ;
#7524=EDGE_LOOP ( 'NONE', ( #12727, #17677, #1738, #18276 ) ) ;
#7537=CARTESIAN_POINT ( 'NONE',  ( 3.943463214271659518E-15, -16.60000000000000142, 22.91316734529526045 ) ) ;
#7549=CIRCLE ( 'NONE', #8444, 5.000000000000004441 ) ;
#7578=ORIENTED_EDGE ( 'NONE', *, *, #11083, .T. ) ;
#7602=AXIS2_PLACEMENT_3D ( 'NONE', #12728, #16757, #18555 ) ;
#7624=VECTOR ( 'NONE', #2588, 1000.000000000000000 ) ;
#7625=VERTEX_POINT ( 'NONE', #4584 ) ;
#7626=EDGE_LOOP ( 'NONE', ( #8783, #8005, #10042, #12268 ) ) ;
#7629=CIRCLE ( 'NONE', #3016, 4.000000000000000000 ) ;
#7632=DIRECTION ( 'NONE',  ( 0.000000000000000000, 0.000000000000000000, -1.000000000000000000 ) ) ;
#7633=CARTESIAN_POINT ( 'NONE',  ( -1.979226605763932723, -19.99999999999999645, 6.000000000000000000 ) ) ;
#7640=ADVANCED_FACE ( 'NONE', ( #14512 ), #14699, .F. ) ;
#7641=FACE_OUTER_BOUND ( 'NONE', #3291, .T. ) ;
#7705=DIRECTION ( 'NONE',  ( 0.000000000000000000, 0.000000000000000000, 1.000000000000000000 ) ) ;
#7737=AXIS2_PLACEMENT_3D ( 'NONE', #3182, #2990, #6168 ) ;
#7748=FACE_BOUND ( 'NONE', #1882, .T. ) ;
#7776=AXIS2_PLACEMENT_3D ( 'NONE', #17268, #17176, #18607 ) ;
#7855=EDGE_CURVE ( 'NONE', #9430, #15279, #13556, .T. ) ;
#7879=VECTOR ( 'NONE', #12530, 1000.000000000000000 ) ;
#7887=ORIENTED_EDGE ( 'NONE', *, *, #15281, .T. ) ;
#7903=DIRECTION ( 'NONE',  ( 0.000000000000000000, 0.000000000000000000, 1.000000000000000000 ) ) ;
#7919=ORIENTED_EDGE ( 'NONE', *, *, #14022, .F. ) ;
#7937=ORIENTED_EDGE ( 'NONE', *, *, #6846, .F. ) ;
#7943=DIRECTION ( 'NONE',  ( 0.000000000000000000, -0.000000000000000000, -1.000000000000000000 ) ) ;
#7944=ORIENTED_EDGE ( 'NONE', *, *, #6802, .T. ) ;
#8005=ORIENTED_EDGE ( 'NONE', *, *, #17474, .T. ) ;
#8011=DIRECTION ( 'NONE',  ( 0.000000000000000000, 0.000000000000000000, -1.000000000000000000 ) ) ;
#8053=DIRECTION ( 'NONE',  ( -0.000000000000000000, 1.000000000000000000, -0.000000000000000000 ) ) ;
#8064=CARTESIAN_POINT ( 'NONE',  ( -194.9999999999999716, -5.000000000000024869, 6.000000000000000000 ) ) ;
#8084=CARTESIAN_POINT ( 'NONE',  ( 4.336808689942017736E-15, -30.00000000000000000, 26.00000000000000000 ) ) ;
#8094=ORIENTED_EDGE ( 'NONE', *, *, #12513, .F. ) ;
#8102=VECTOR ( 'NONE', #17735, 1000.000000000000000 ) ;
#8155=CARTESIAN_POINT ( 'NONE',  ( 0.000000000000000000, 0.000000000000000000, 6.000000000000000000 ) ) ;
#8183=ORIENTED_EDGE ( 'NONE', *, *, #847, .T. ) ;
#8186=EDGE_LOOP ( 'NONE', ( #2078, #12409, #2652, #7000 ) ) ;
#8187=VECTOR ( 'NONE', #17538, 1000.000000000000000 ) ;
#8191=ADVANCED_FACE ( 'NONE', ( #7268 ), #16146, .F. ) ;
#8236=STYLED_ITEM ( 'NONE', ( #4920 ), #3553 ) ;
#8249=LINE ( 'NONE', #3935, #7879 ) ;
#8275=ORIENTED_EDGE ( 'NONE', *, *, #3603, .T. ) ;
#8282=( NAMED_UNIT ( * ) PLANE_ANGLE_UNIT ( ) SI_UNIT ( $, .RADIAN. ) );
#8334=CARTESIAN_POINT ( 'NONE',  ( -58.82978549640777288, -10.68512861272757952, 3.000000000000000000 ) ) ;
#8337=FACE_BOUND ( 'NONE', #10112, .T. ) ;
#8342=ADVANCED_FACE ( 'NONE', ( #578, #11943 ), #4963, .F. ) ;
#8344=VERTEX_POINT ( 'NONE', #1813 ) ;
#8354=LINE ( 'NONE', #2595, #14273 ) ;
#8357=LINE ( 'NONE', #14361, #5098 ) ;
#8367=ADVANCED_FACE ( 'NONE', ( #12141 ), #13462, .F. ) ;
#8393=FACE_BOUND ( 'NONE', #17147, .T. ) ;
#8433=CARTESIAN_POINT ( 'NONE',  ( 3.686287386450715076E-15, -16.60000000000000142, 21.01316734529526187 ) ) ;
#8436=EDGE_CURVE ( 'NONE', #9382, #3145, #5145, .T. ) ;
#8444=AXIS2_PLACEMENT_3D ( 'NONE', #2394, #7085, #6804 ) ;
#8449=CIRCLE ( 'NONE', #18824, 5.000000000000000888 ) ;
#8487=VECTOR ( 'NONE', #858, 1000.000000000000000 ) ;
#8493=ORIENTED_EDGE ( 'NONE', *, *, #15182, .T. ) ;
#8495=FACE_OUTER_BOUND ( 'NONE', #2077, .T. ) ;
#8501=CARTESIAN_POINT ( 'NONE',  ( -1.979226605763932723, -14.99999999999999645, 6.000000000000000000 ) ) ;
#8506=DIRECTION ( 'NONE',  ( -1.000000000000000000, -5.782411586589358625E-16, 0.000000000000000000 ) ) ;
#8521=EDGE_LOOP ( 'NONE', ( #6243, #17096, #6694, #13724 ) ) ;
#8539=ORIENTED_EDGE ( 'NONE', *, *, #2491, .F. ) ;
#8547=ORIENTED_EDGE ( 'NONE', *, *, #17014, .F. ) ;
#8553=DIRECTION ( 'NONE',  ( 0.000000000000000000, 0.000000000000000000, 1.000000000000000000 ) ) ;
#8575=EDGE_CURVE ( 'NONE', #18014, #14303, #11350, .T. ) ;
#8581=ORIENTED_EDGE ( 'NONE', *, *, #6846, .T. ) ;
#8604=CYLINDRICAL_SURFACE ( 'NONE', #16898, 5.000000000000000000 ) ;
#8615=ORIENTED_EDGE ( 'NONE', *, *, #2528, .F. ) ;
#8623=CARTESIAN_POINT ( 'NONE',  ( -194.9999999999999716, 9.999999999999973355, 6.000000000000000000 ) ) ;
#8646=EDGE_CURVE ( 'NONE', #13406, #12130, #18036, .T. ) ;
#8654=ORIENTED_EDGE ( 'NONE', *, *, #11834, .T. ) ;
#8679=CIRCLE ( 'NONE', #2902, 5.000000000000000888 ) ;
#8744=DIRECTION ( 'NONE',  ( 0.000000000000000000, 1.000000000000000000, 0.000000000000000000 ) ) ;
#8745=FACE_OUTER_BOUND ( 'NONE', #4454, .T. ) ;
#8759=ADVANCED_FACE ( 'NONE', ( #14968 ), #10684, .F. ) ;
#8783=ORIENTED_EDGE ( 'NONE', *, *, #2654, .F. ) ;
#8832=CARTESIAN_POINT ( 'NONE',  ( -194.9999999999999716, 4.999999999999973355, 6.000000000000000000 ) ) ;
#8836=FACE_OUTER_BOUND ( 'NONE', #13635, .T. ) ;
#8837=CARTESIAN_POINT ( 'NONE',  ( 1.136782529653004747, -40.00000000000000000, 6.000000000000000000 ) ) ;
#8843=ORIENTED_EDGE ( 'NONE', *, *, #2244, .F. ) ;
#8856=DIRECTION ( 'NONE',  ( -0.000000000000000000, -0.000000000000000000, 1.000000000000000000 ) ) ;
#8873=CARTESIAN_POINT ( 'NONE',  ( 20.00000000000000711, -45.00000000000000000, 6.000000000000000000 ) ) ;
#8893=DIRECTION ( 'NONE',  ( -1.000000000000000000, 0.000000000000000000, 0.000000000000000000 ) ) ;
#8898=DIRECTION ( 'NONE',  ( 0.000000000000000000, 0.000000000000000000, -1.000000000000000000 ) ) ;
#8923=CARTESIAN_POINT ( 'NONE',  ( 3.686287386450715076E-15, -16.60000000000000142, 25.01316734529526187 ) ) ;
#8925=LINE ( 'NONE', #14853, #2918 ) ;
#8926=CARTESIAN_POINT ( 'NONE',  ( -55.93192566395838128, 4.999999999999974243, 3.000000000000000000 ) ) ;
#8948=EDGE_CURVE ( 'NONE', #11387, #846, #4456, .T. ) ;
#8998=VECTOR ( 'NONE', #355, 1000.000000000000000 ) ;
#9009=CARTESIAN_POINT ( 'NONE',  ( 20.00000000000000711, -24.99999999999999645, 6.000000000000000000 ) ) ;
#9013=VECTOR ( 'NONE', #2059, 1000.000000000000000 ) ;
#9036=LINE ( 'NONE', #11709, #8187 ) ;
#9061=AXIS2_PLACEMENT_3D ( 'NONE', #8837, #12092, #1868 ) ;
#9078=EDGE_CURVE ( 'NONE', #11185, #182, #8925, .T. ) ;
#9103=ADVANCED_FACE ( 'NONE', ( #8836 ), #1963, .F. ) ;
#9130=DIRECTION ( 'NONE',  ( -0.000000000000000000, -0.000000000000000000, 1.000000000000000000 ) ) ;
#9216=DIRECTION ( 'NONE',  ( -0.000000000000000000, 1.000000000000000000, -0.000000000000000000 ) ) ;
#9221=CARTESIAN_POINT ( 'NONE',  ( 15.00000000000000711, -45.00000000000000000, 3.000000000000000000 ) ) ;
#9240=CARTESIAN_POINT ( 'NONE',  ( -30.00000000000000355, -12.50000000000000178, 3.000000000000000000 ) ) ;
#9265=EDGE_CURVE ( 'NONE', #15782, #3563, #18770, .T. ) ;
#9277=VECTOR ( 'NONE', #11631, 1000.000000000000000 ) ;
#9288=AXIS2_PLACEMENT_3D ( 'NONE', #13021, #1180, #3958 ) ;
#9289=EDGE_CURVE ( 'NONE', #13349, #14649, #6735, .T. ) ;
#9315=CARTESIAN_POINT ( 'NONE',  ( -194.9999999999999716, -10.00000000000002665, 6.000000000000000000 ) ) ;
#9333=ORIENTED_EDGE ( 'NONE', *, *, #11989, .T. ) ;
#9356=VERTEX_POINT ( 'NONE', #11590 ) ;
#9371=EDGE_LOOP ( 'NONE', ( #10290, #16530 ) ) ;
#9381=AXIS2_PLACEMENT_3D ( 'NONE', #9829, #8053, #13774 ) ;
#9382=VERTEX_POINT ( 'NONE', #15687 ) ;
#9391=AXIS2_PLACEMENT_3D ( 'NONE', #8155, #1056, #6898 ) ;
#9396=CYLINDRICAL_SURFACE ( 'NONE', #15189, 5.000000000000004441 ) ;
#9397=CIRCLE ( 'NONE', #15497, 4.999999999999997335 ) ;
#9430=VERTEX_POINT ( 'NONE', #3055 ) ;
#9499=LINE ( 'NONE', #6364, #12129 ) ;
#9575=ORIENTED_EDGE ( 'NONE', *, *, #8646, .F. ) ;
#9580=VERTEX_POINT ( 'NONE', #6523 ) ;
#9582=CARTESIAN_POINT ( 'NONE',  ( -55.93192566395838128, 4.999999999999974243, 6.000000000000000000 ) ) ;
#9594=PLANE ( 'NONE',  #2647 ) ;
#9680=CIRCLE ( 'NONE', #3881, 2.100000000000000977 ) ;
#9700=ORIENTED_EDGE ( 'NONE', *, *, #11989, .F. ) ;
#9710=CARTESIAN_POINT ( 'NONE',  ( -53.40568638168567617, 9.314871387272406267, 6.000000000000000000 ) ) ;
#9724=EDGE_LOOP ( 'NONE', ( #10698, #3246, #15938, #1590, #656, #262, #516, #8183, #4175, #6661, #14693, #1903, #3986, #17863, #15608, #4377 ) ) ;
#9772=CYLINDRICAL_SURFACE ( 'NONE', #17508, 2.499999999999992006 ) ;
#9778=EDGE_CURVE ( 'NONE', #182, #9430, #13292, .T. ) ;
#9829=CARTESIAN_POINT ( 'NONE',  ( 4.336808689942017736E-15, -27.00000000000000000, 26.00000000000000000 ) ) ;
#9832=DIRECTION ( 'NONE',  ( 0.000000000000000000, 0.000000000000000000, -1.000000000000000000 ) ) ;
#9834=CARTESIAN_POINT ( 'NONE',  ( 3.686287386450715076E-15, -27.00000000000000000, 27.11316734529526329 ) ) ;
#9850=LINE ( 'NONE', #17506, #6080 ) ;
#9908=CARTESIAN_POINT ( 'NONE',  ( -199.9999999999999716, 4.999999999999973355, 3.000000000000000000 ) ) ;
#9975=CLOSED_SHELL ( 'NONE', ( #268, #5734, #5724, #3915, #15600, #10576, #976, #8191, #7640, #9103, #1869, #17348, #5924, #624, #12284, #11780, #18836, #3755, #8367, #3695, #5010, #3521, #15514, #8759, #8342, #18886, #17901, #13855, #1890, #18741, #4957, #11858, #10075 ) ) ;
#9987=EDGE_LOOP ( 'NONE', ( #18767, #14407, #16907, #1519, #11725, #10140, #6752, #15273, #12559, #7307, #8094, #840, #6793, #12909, #3445, #14720 ) ) ;
#10015=VERTEX_POINT ( 'NONE', #11152 ) ;
#10023=DIRECTION ( 'NONE',  ( 0.000000000000000000, 0.000000000000000000, 1.000000000000000000 ) ) ;
#10038=CARTESIAN_POINT ( 'NONE',  ( 5.000000000000006217, -30.00000000000000000, 26.00000000000000000 ) ) ;
#10041=AXIS2_PLACEMENT_3D ( 'NONE', #8832, #5957, #17166 ) ;
#10042=ORIENTED_EDGE ( 'NONE', *, *, #17360, .T. ) ;
#10053=AXIS2_PLACEMENT_3D ( 'NONE', #4498, #4590, #13467 ) ;
#10069=DIRECTION ( 'NONE',  ( 0.000000000000000000, 0.000000000000000000, -1.000000000000000000 ) ) ;
#10075=ADVANCED_FACE ( 'NONE', ( #8745 ), #5647, .F. ) ;
#10094=CARTESIAN_POINT ( 'NONE',  ( -32.49999999999999289, -12.50000000000000178, 6.000000000000000000 ) ) ;
#10112=EDGE_LOOP ( 'NONE', ( #15272, #6833, #17966, #15582 ) ) ;
#10124=PLANE ( 'NONE',  #4113 ) ;
#10125=CARTESIAN_POINT ( 'NONE',  ( -4.999999999999995559, -27.00000000000000000, 6.000000000000000000 ) ) ;
#10140=ORIENTED_EDGE ( 'NONE', *, *, #11103, .T. ) ;
#10156=DIRECTION ( 'NONE',  ( 1.000000000000000000, 0.000000000000000000, 0.000000000000000000 ) ) ;
#10169=VECTOR ( 'NONE', #2262, 1000.000000000000000 ) ;
#10186=VERTEX_POINT ( 'NONE', #1871 ) ;
#10201=CARTESIAN_POINT ( 'NONE',  ( -194.9999999999999716, -10.00000000000002665, 3.000000000000000000 ) ) ;
#10217=DIRECTION ( 'NONE',  ( 0.000000000000000000, -1.000000000000000000, 0.000000000000000000 ) ) ;
#10227=DIRECTION ( 'NONE',  ( -0.000000000000000000, 1.000000000000000000, -0.000000000000000000 ) ) ;
#10279=ORIENTED_EDGE ( 'NONE', *, *, #14843, .F. ) ;
#10290=ORIENTED_EDGE ( 'NONE', *, *, #10925, .F. ) ;
#10319=FACE_OUTER_BOUND ( 'NONE', #7480, .T. ) ;
#10335=UNCERTAINTY_MEASURE_WITH_UNIT (LENGTH_MEASURE( 1.000000000000000082E-05 ), #244, 'distance_accuracy_value', 'NONE');
#10339=CARTESIAN_POINT ( 'NONE',  ( 5.000000000000006217, -30.00000000000000000, 6.000000000000000000 ) ) ;
#10344=ORIENTED_EDGE ( 'NONE', *, *, #15281, .F. ) ;
#10360=VECTOR ( 'NONE', #13563, 1000.000000000000000 ) ;
#10400=EDGE_LOOP ( 'NONE', ( #10279, #18185, #4992, #3260 ) ) ;
#10430=DIRECTION ( 'NONE',  ( 0.000000000000000000, 0.000000000000000000, -1.000000000000000000 ) ) ;
#10474=ORIENTED_EDGE ( 'NONE', *, *, #2695, .F. ) ;
#10501=ORIENTED_EDGE ( 'NONE', *, *, #9265, .T. ) ;
#10507=DIRECTION ( 'NONE',  ( 0.000000000000000000, -0.000000000000000000, -1.000000000000000000 ) ) ;
#10566=COLOUR_RGB ( '', 0.09019608, 0.27058824, 0.51372549) ;
#10576=ADVANCED_FACE ( 'NONE', ( #3995, #8393 ), #5335, .T. ) ;
#10611=DIRECTION ( 'NONE',  ( 0.000000000000000000, 0.000000000000000000, -1.000000000000000000 ) ) ;
#10628=VECTOR ( 'NONE', #1774, 1000.000000000000000 ) ;
#10664=LINE ( 'NONE', #3379, #16944 ) ;
#10684=PLANE ( 'NONE',  #15744 ) ;
#10687=VECTOR ( 'NONE', #13771, 1000.000000000000000 ) ;
#10694=DIRECTION ( 'NONE',  ( -0.000000000000000000, -0.000000000000000000, 1.000000000000000000 ) ) ;
#10698=ORIENTED_EDGE ( 'NONE', *, *, #11591, .T. ) ;
#10749=( LENGTH_UNIT ( ) NAMED_UNIT ( * ) SI_UNIT ( .MILLI., .METRE. ) );
#10752=CIRCLE ( 'NONE', #3414, 2.499999999999995115 ) ;
#10773=CARTESIAN_POINT ( 'NONE',  ( -4.505465888036638944, -19.31487138727242225, 3.000000000000000000 ) ) ;
#10781=DIRECTION ( 'NONE',  ( -1.000000000000000000, 0.000000000000000000, 0.000000000000000000 ) ) ;
#10832=LINE ( 'NONE', #5082, #3402 ) ;
#10859=AXIS2_PLACEMENT_3D ( 'NONE', #12459, #16853, #12633 ) ;
#10882=CARTESIAN_POINT ( 'NONE',  ( -1.979226605763932723, -19.99999999999999645, 3.000000000000000000 ) ) ;
#10886=DIRECTION ( 'NONE',  ( 0.000000000000000000, 0.000000000000000000, -1.000000000000000000 ) ) ;
#10890=ORIENTED_EDGE ( 'NONE', *, *, #16666, .F. ) ;
#10901=EDGE_LOOP ( 'NONE', ( #18875, #12109, #553 ) ) ;
#10924=DIRECTION ( 'NONE',  ( -1.000000000000000000, 0.000000000000000000, 0.000000000000000000 ) ) ;
#10925=EDGE_CURVE ( 'NONE', #2805, #10015, #4059, .T. ) ;
#10972=CYLINDRICAL_SURFACE ( 'NONE', #11166, 5.000000000000000888 ) ;
#11068=LINE ( 'NONE', #5225, #14865 ) ;
#11083=EDGE_CURVE ( 'NONE', #12603, #15726, #5873, .T. ) ;
#11103=EDGE_CURVE ( 'NONE', #14649, #998, #3444, .T. ) ;
#11117=EDGE_LOOP ( 'NONE', ( #14489, #8581, #1978, #10344 ) ) ;
#11147=CARTESIAN_POINT ( 'NONE',  ( -55.93192566395838128, 9.999999999999973355, 6.000000000000000000 ) ) ;
#11152=CARTESIAN_POINT ( 'NONE',  ( 4.176146106109656457E-15, -16.60000000000000142, 29.01316734529526187 ) ) ;
#11153=VECTOR ( 'NONE', #17201, 1000.000000000000000 ) ;
#11166=AXIS2_PLACEMENT_3D ( 'NONE', #5130, #8011, #10781 ) ;
#11185=VERTEX_POINT ( 'NONE', #9221 ) ;
#11187=CARTESIAN_POINT ( 'NONE',  ( 3.686287386450715076E-15, -16.60000000000000142, 25.01316734529526187 ) ) ;
#11227=LINE ( 'NONE', #15595, #7314 ) ;
#11241=ORIENTED_EDGE ( 'NONE', *, *, #1285, .F. ) ;
#11248=DIRECTION ( 'NONE',  ( 0.000000000000000000, 0.000000000000000000, 1.000000000000000000 ) ) ;
#11293=CARTESIAN_POINT ( 'NONE',  ( 15.00000000000000711, -40.00000000000000000, 6.000000000000000000 ) ) ;
#11314=UNCERTAINTY_MEASURE_WITH_UNIT (LENGTH_MEASURE( 1.000000000000000082E-05 ), #10749, 'distance_accuracy_value', 'NONE');
#11342=LINE ( 'NONE', #6951, #14543 ) ;
#11349=CYLINDRICAL_SURFACE ( 'NONE', #10041, 5.000000000000004441 ) ;
#11350=LINE ( 'NONE', #10094, #190 ) ;
#11369=EDGE_LOOP ( 'NONE', ( #16134, #1190, #8654, #5478 ) ) ;
#11387=VERTEX_POINT ( 'NONE', #8623 ) ;
#11419=VECTOR ( 'NONE', #17382, 1000.000000000000000 ) ;
#11425=DIRECTION ( 'NONE',  ( 0.000000000000000000, 0.000000000000000000, -1.000000000000000000 ) ) ;
#11452=LINE ( 'NONE', #14502, #6324 ) ;
#11512=CIRCLE ( 'NONE', #17937, 2.499999999999995115 ) ;
#11538=DIRECTION ( 'NONE',  ( -0.000000000000000000, -0.000000000000000000, -1.000000000000000000 ) ) ;
#11555=ORIENTED_EDGE ( 'NONE', *, *, #9778, .F. ) ;
#11560=LINE ( 'NONE', #17283, #11419 ) ;
#11564=DIRECTION ( 'NONE',  ( 0.000000000000000000, -0.000000000000000000, -1.000000000000000000 ) ) ;
#11590=CARTESIAN_POINT ( 'NONE',  ( 1.136782529653004747, -45.00000000000000000, 3.000000000000000000 ) ) ;
#11591=EDGE_CURVE ( 'NONE', #10186, #18408, #3457, .T. ) ;
#11619=DIRECTION ( 'NONE',  ( -0.000000000000000000, -0.000000000000000000, 1.000000000000000000 ) ) ;
#11631=DIRECTION ( 'NONE',  ( -0.000000000000000000, -1.000000000000000000, -0.000000000000000000 ) ) ;
#11633=LINE ( 'NONE', #7537, #13415 ) ;
#11657=DIRECTION ( 'NONE',  ( -5.782411586589358625E-16, 1.000000000000000000, 0.000000000000000000 ) ) ;
#11663=DIRECTION ( 'NONE',  ( 0.000000000000000000, 0.000000000000000000, 1.000000000000000000 ) ) ;
#11665=AXIS2_PLACEMENT_3D ( 'NONE', #1419, #7163, #12975 ) ;
#11669=CARTESIAN_POINT ( 'NONE',  ( 3.943463214271659518E-15, -27.00000000000000000, 22.91316734529526045 ) ) ;
#11676=LINE ( 'NONE', #1254, #5106 ) ;
#11680=AXIS2_PLACEMENT_3D ( 'NONE', #14379, #6760, #5406 ) ;
#11689=EDGE_CURVE ( 'NONE', #1651, #3145, #2216, .T. ) ;
#11693=DIRECTION ( 'NONE',  ( -1.000000000000000000, 0.000000000000000000, 0.000000000000000000 ) ) ;
#11707=SURFACE_SIDE_STYLE ('',( #4350 ) ) ;
#11709=CARTESIAN_POINT ( 'NONE',  ( 1.136782529653004747, -45.00000000000000000, 6.000000000000000000 ) ) ;
#11725=ORIENTED_EDGE ( 'NONE', *, *, #17877, .F. ) ;
#11780=ADVANCED_FACE ( 'NONE', ( #1336 ), #8604, .T. ) ;
#11810=VECTOR ( 'NONE', #12283, 1000.000000000000000 ) ;
#11817=AXIS2_PLACEMENT_3D ( 'NONE', #8926, #13323, #13420 ) ;
#11834=EDGE_CURVE ( 'NONE', #15279, #1391, #4306, .T. ) ;
#11856=CARTESIAN_POINT ( 'NONE',  ( 1.136782529653004747, -40.00000000000000000, 6.000000000000000000 ) ) ;
#11858=ADVANCED_FACE ( 'NONE', ( #1441 ), #13092, .F. ) ;
#11872=DIRECTION ( 'NONE',  ( 0.000000000000000000, 0.000000000000000000, -1.000000000000000000 ) ) ;
#11892=AXIS2_PLACEMENT_3D ( 'NONE', #9582, #8898, #4322 ) ;
#11904=DIRECTION ( 'NONE',  ( 0.000000000000000000, 0.000000000000000000, -1.000000000000000000 ) ) ;
#11932=APPLICATION_CONTEXT ( 'automotive_design' ) ;
#11933=ORIENTED_EDGE ( 'NONE', *, *, #5439, .F. ) ;
#11943=FACE_OUTER_BOUND ( 'NONE', #1605, .T. ) ;
#11956=CARTESIAN_POINT ( 'NONE',  ( -61.35602477868047799, -15.00000000000000711, 3.000000000000000000 ) ) ;
#11989=EDGE_CURVE ( 'NONE', #15782, #1651, #3696, .T. ) ;
#12009=ORIENTED_EDGE ( 'NONE', *, *, #13925, .T. ) ;
#12011=EDGE_LOOP ( 'NONE', ( #4453, #18528, #255, #15888 ) ) ;
#12012=CARTESIAN_POINT ( 'NONE',  ( 20.00000000000000711, -24.99999999999999645, 3.000000000000000000 ) ) ;
#12053=DIRECTION ( 'NONE',  ( -1.000000000000000000, 3.469446951953611033E-15, 0.000000000000000000 ) ) ;
#12092=DIRECTION ( 'NONE',  ( -0.000000000000000000, -0.000000000000000000, 1.000000000000000000 ) ) ;
#12105=EDGE_LOOP ( 'NONE', ( #14049, #15733, #16643, #15080 ) ) ;
#12109=ORIENTED_EDGE ( 'NONE', *, *, #17014, .T. ) ;
#12113=DIRECTION ( 'NONE',  ( 5.782411586589358625E-16, -1.000000000000000000, 0.000000000000000000 ) ) ;
#12129=VECTOR ( 'NONE', #3480, 1000.000000000000000 ) ;
#12130=VERTEX_POINT ( 'NONE', #14956 ) ;
#12140=CARTESIAN_POINT ( 'NONE',  ( 3.686287386450715076E-15, -16.60000000000000142, 25.01316734529526187 ) ) ;
#12141=FACE_OUTER_BOUND ( 'NONE', #282, .T. ) ;
#12160=CARTESIAN_POINT ( 'NONE',  ( 15.00000000000000711, -24.99999999999999645, 3.000000000000000000 ) ) ;
#12233=DIRECTION ( 'NONE',  ( 0.000000000000000000, 0.000000000000000000, 1.000000000000000000 ) ) ;
#12247=CARTESIAN_POINT ( 'NONE',  ( -4.999999999999995559, -27.00000000000000000, 31.00000000000000000 ) ) ;
#12268=ORIENTED_EDGE ( 'NONE', *, *, #3271, .F. ) ;
#12278=PRODUCT ( 'Handle arm 2', 'Handle arm 2', '', ( #3671 ) ) ;
#12283=DIRECTION ( 'NONE',  ( -0.000000000000000000, -0.000000000000000000, 1.000000000000000000 ) ) ;
#12284=ADVANCED_FACE ( 'NONE', ( #6744 ), #9772, .F. ) ;
#12409=ORIENTED_EDGE ( 'NONE', *, *, #15117, .T. ) ;
#12434=ORIENTED_EDGE ( 'NONE', *, *, #15204, .T. ) ;
#12459=CARTESIAN_POINT ( 'NONE',  ( 6.071532165918821675E-15, -30.00000000000000000, 26.00000000000000000 ) ) ;
#12473=ORIENTED_EDGE ( 'NONE', *, *, #17273, .F. ) ;
#12495=CIRCLE ( 'NONE', #4264, 5.000000000000000000 ) ;
#12508=EDGE_LOOP ( 'NONE', ( #3251, #5481, #16465, #14125 ) ) ;
#12513=EDGE_CURVE ( 'NONE', #12130, #15007, #10832, .T. ) ;
#12519=FACE_OUTER_BOUND ( 'NONE', #10400, .T. ) ;
#12527=DIRECTION ( 'NONE',  ( 0.000000000000000000, 0.000000000000000000, -1.000000000000000000 ) ) ;
#12530=DIRECTION ( 'NONE',  ( -0.000000000000000000, -1.000000000000000000, -0.000000000000000000 ) ) ;
#12555=CARTESIAN_POINT ( 'NONE',  ( 20.00000000000000711, -40.00000000000000000, 3.000000000000000000 ) ) ;
#12556=VECTOR ( 'NONE', #12527, 1000.000000000000000 ) ;
#12559=ORIENTED_EDGE ( 'NONE', *, *, #1919, .F. ) ;
#12597=ORIENTED_EDGE ( 'NONE', *, *, #3757, .F. ) ;
#12603=VERTEX_POINT ( 'NONE', #5535 ) ;
#12633=DIRECTION ( 'NONE',  ( 0.000000000000000000, 0.000000000000000000, 1.000000000000000000 ) ) ;
#12638=EDGE_CURVE ( 'NONE', #13171, #13464, #15399, .T. ) ;
#12648=VECTOR ( 'NONE', #14611, 1000.000000000000000 ) ;
#12673=VERTEX_POINT ( 'NONE', #8334 ) ;
#12674=AXIS2_PLACEMENT_3D ( 'NONE', #2988, #15908, #8553 ) ;
#12681=DIRECTION ( 'NONE',  ( -0.000000000000000000, -0.000000000000000000, -1.000000000000000000 ) ) ;
#12711=DIRECTION ( 'NONE',  ( -1.000000000000000000, 1.387778780781445478E-15, 0.000000000000000000 ) ) ;
#12713=AXIS2_PLACEMENT_3D ( 'NONE', #11187, #13143, #7331 ) ;
#12714=CIRCLE ( 'NONE', #17610, 5.000000000000000888 ) ;
#12727=ORIENTED_EDGE ( 'NONE', *, *, #18129, .F. ) ;
#12728=CARTESIAN_POINT ( 'NONE',  ( -194.9999999999999716, -5.000000000000024869, 6.000000000000000000 ) ) ;
#12801=CARTESIAN_POINT ( 'NONE',  ( -199.9999999999999716, 9.999999999999973355, 3.000000000000000000 ) ) ;
#12844=DIRECTION ( 'NONE',  ( 0.000000000000000000, -1.000000000000000000, 0.000000000000000000 ) ) ;
#12909=ORIENTED_EDGE ( 'NONE', *, *, #581, .T. ) ;
#12914=LINE ( 'NONE', #17411, #17699 ) ;
#12975=DIRECTION ( 'NONE',  ( 0.000000000000000000, 0.000000000000000000, -1.000000000000000000 ) ) ;
#12984=CARTESIAN_POINT ( 'NONE',  ( -1.127570259384925242E-14, -6.520075332560959849E-30, 26.00000000000000000 ) ) ;
#13021=CARTESIAN_POINT ( 'NONE',  ( -61.35602477868047799, -15.00000000000000711, 6.000000000000000000 ) ) ;
#13041=SHAPE_REPRESENTATION_RELATIONSHIP ( 'NONE' , 'NONE' ,  #5797, #18114 ) ;
#13071=ORIENTED_EDGE ( 'NONE', *, *, #9289, .F. ) ;
#13076=CARTESIAN_POINT ( 'NONE',  ( -199.9999999999999716, 4.999999999999973355, 6.000000000000000000 ) ) ;
#13092=CYLINDRICAL_SURFACE ( 'NONE', #1009, 2.100000000000000977 ) ;
#13104=EDGE_LOOP ( 'NONE', ( #6062, #552, #3113, #2605 ) ) ;
#13143=DIRECTION ( 'NONE',  ( 0.000000000000000000, -1.000000000000000000, 0.000000000000000000 ) ) ;
#13168=EDGE_LOOP ( 'NONE', ( #3980, #13813, #9333, #15187 ) ) ;
#13171=VERTEX_POINT ( 'NONE', #647 ) ;
#13172=CARTESIAN_POINT ( 'NONE',  ( -199.9999999999999716, -5.000000000000024869, 3.000000000000000000 ) ) ;
#13226=DIRECTION ( 'NONE',  ( -0.5052478564545411777, -0.8629742774544855166, 0.000000000000000000 ) ) ;
#13255=CARTESIAN_POINT ( 'NONE',  ( 15.00000000000000711, -19.99999999999999645, 3.000000000000000000 ) ) ;
#13257=VERTEX_POINT ( 'NONE', #2280 ) ;
#13292=CIRCLE ( 'NONE', #14208, 5.000000000000000888 ) ;
#13295=EDGE_LOOP ( 'NONE', ( #11933, #18060, #18878, #5327 ) ) ;
#13323=DIRECTION ( 'NONE',  ( 0.000000000000000000, 0.000000000000000000, -1.000000000000000000 ) ) ;
#13325=DIRECTION ( 'NONE',  ( 0.000000000000000000, 0.000000000000000000, -1.000000000000000000 ) ) ;
#13328=DIRECTION ( 'NONE',  ( -0.000000000000000000, 1.000000000000000000, -0.000000000000000000 ) ) ;
#13329=CYLINDRICAL_SURFACE ( 'NONE', #2371, 5.000000000000000888 ) ;
#13349=VERTEX_POINT ( 'NONE', #5600 ) ;
#13370=FACE_OUTER_BOUND ( 'NONE', #9371, .T. ) ;
#13406=VERTEX_POINT ( 'NONE', #1216 ) ;
#13415=VECTOR ( 'NONE', #14881, 1000.000000000000000 ) ;
#13420=DIRECTION ( 'NONE',  ( -1.000000000000000000, 0.000000000000000000, 0.000000000000000000 ) ) ;
#13462=CYLINDRICAL_SURFACE ( 'NONE', #3841, 5.000000000000000000 ) ;
#13464=VERTEX_POINT ( 'NONE', #13255 ) ;
#13467=DIRECTION ( 'NONE',  ( 0.000000000000000000, 0.000000000000000000, -1.000000000000000000 ) ) ;
#13480=CARTESIAN_POINT ( 'NONE',  ( 1.136782529653004747, -45.00000000000000000, 6.000000000000000000 ) ) ;
#13493=CARTESIAN_POINT ( 'NONE',  ( -0.2192422490275049152, -45.00000000000000000, 6.000000000000000000 ) ) ;
#13554=CIRCLE ( 'NONE', #4384, 2.499999999999995115 ) ;
#13556=LINE ( 'NONE', #16441, #16640 ) ;
#13563=DIRECTION ( 'NONE',  ( 1.000000000000000000, -0.000000000000000000, -0.000000000000000000 ) ) ;
#13577=AXIS2_PLACEMENT_3D ( 'NONE', #8873, #1809, #87 ) ;
#13612=DIRECTION ( 'NONE',  ( 0.000000000000000000, 0.000000000000000000, -1.000000000000000000 ) ) ;
#13635=EDGE_LOOP ( 'NONE', ( #2724, #17768, #4577, #18341 ) ) ;
#13681=VECTOR ( 'NONE', #15619, 1000.000000000000000 ) ;
#13711=DIRECTION ( 'NONE',  ( -0.000000000000000000, 1.000000000000000000, -0.000000000000000000 ) ) ;
#13724=ORIENTED_EDGE ( 'NONE', *, *, #14910, .T. ) ;
#13730=EDGE_LOOP ( 'NONE', ( #5398, #5212, #3493, #994 ) ) ;
#13748=EDGE_CURVE ( 'NONE', #15007, #8344, #1289, .T. ) ;
#13771=DIRECTION ( 'NONE',  ( 1.000000000000000000, 0.000000000000000000, 0.000000000000000000 ) ) ;
#13774=DIRECTION ( 'NONE',  ( 0.000000000000000000, 0.000000000000000000, -1.000000000000000000 ) ) ;
#13785=ORIENTED_EDGE ( 'NONE', *, *, #10925, .T. ) ;
#13813=ORIENTED_EDGE ( 'NONE', *, *, #2695, .T. ) ;
#13855=ADVANCED_FACE ( 'NONE', ( #4548 ), #13329, .T. ) ;
#13888=CARTESIAN_POINT ( 'NONE',  ( 3.686287386450715076E-15, -27.00000000000000000, 25.01316734529526187 ) ) ;
#13913=FACE_OUTER_BOUND ( 'NONE', #1942, .T. ) ;
#13925=EDGE_CURVE ( 'NONE', #6600, #9356, #9036, .T. ) ;
#13939=CIRCLE ( 'NONE', #2939, 4.000000000000000000 ) ;
#13945=EDGE_CURVE ( 'NONE', #1518, #11387, #1578, .T. ) ;
#13950=AXIS2_PLACEMENT_3D ( 'NONE', #904, #18385, #2504 ) ;
#13981=CARTESIAN_POINT ( 'NONE',  ( -194.9999999999999716, 9.999999999999973355, 3.000000000000000000 ) ) ;
#14003=CIRCLE ( 'NONE', #14744, 5.000000000000000000 ) ;
#14022=EDGE_CURVE ( 'NONE', #8344, #13257, #9397, .T. ) ;
#14049=ORIENTED_EDGE ( 'NONE', *, *, #17474, .F. ) ;
#14097=DIRECTION ( 'NONE',  ( 0.000000000000000000, 0.000000000000000000, -1.000000000000000000 ) ) ;
#14100=CIRCLE ( 'NONE', #11665, 5.000000000000000888 ) ;
#14124=EDGE_CURVE ( 'NONE', #12130, #18846, #3906, .T. ) ;
#14125=ORIENTED_EDGE ( 'NONE', *, *, #4769, .F. ) ;
#14147=EDGE_CURVE ( 'NONE', #13349, #5705, #8354, .T. ) ;
#14150=CARTESIAN_POINT ( 'NONE',  ( -194.9999999999999716, 4.999999999999973355, 3.000000000000000000 ) ) ;
#14162=CARTESIAN_POINT ( 'NONE',  ( 20.00000000000000711, -45.00000000000000000, 3.000000000000000000 ) ) ;
#14171=DIRECTION ( 'NONE',  ( 1.000000000000000000, 1.239088197126290570E-16, -0.000000000000000000 ) ) ;
#14208=AXIS2_PLACEMENT_3D ( 'NONE', #11293, #1238, #12711 ) ;
#14219=CARTESIAN_POINT ( 'NONE',  ( -4.999999999999995559, -30.00000000000000000, 6.000000000000000000 ) ) ;
#14221=CARTESIAN_POINT ( 'NONE',  ( 5.000000000000004441, -27.00000000000000000, 6.000000000000000000 ) ) ;
#14240=LINE ( 'NONE', #12801, #12648 ) ;
#14273=VECTOR ( 'NONE', #14171, 1000.000000000000000 ) ;
#14292=EDGE_CURVE ( 'NONE', #13464, #18846, #2199, .T. ) ;
#14303=VERTEX_POINT ( 'NONE', #18254 ) ;
#14322=CYLINDRICAL_SURFACE ( 'NONE', #12713, 4.000000000000000000 ) ;
#14334=LINE ( 'NONE', #10125, #5759 ) ;
#14337=LINE ( 'NONE', #18720, #11153 ) ;
#14361=CARTESIAN_POINT ( 'NONE',  ( -27.50000000000000711, -12.50000000000000178, 6.000000000000000000 ) ) ;
#14370=VERTEX_POINT ( 'NONE', #9009 ) ;
#14375=APPLICATION_CONTEXT ( 'automotive_design' ) ;
#14379=CARTESIAN_POINT ( 'NONE',  ( 3.686287386450715076E-15, -16.60000000000000142, 25.01316734529526187 ) ) ;
#14387=ORIENTED_EDGE ( 'NONE', *, *, #1285, .T. ) ;
#14407=ORIENTED_EDGE ( 'NONE', *, *, #85, .T. ) ;
#14419=DIRECTION ( 'NONE',  ( -1.000000000000000000, -0.000000000000000000, -0.000000000000000000 ) ) ;
#14469=FACE_OUTER_BOUND ( 'NONE', #3817, .T. ) ;
#14489=ORIENTED_EDGE ( 'NONE', *, *, #15204, .F. ) ;
#14502=CARTESIAN_POINT ( 'NONE',  ( -3.335251384444446021, -19.99999999999999645, 6.000000000000000000 ) ) ;
#14512=FACE_OUTER_BOUND ( 'NONE', #13104, .T. ) ;
#14518=VECTOR ( 'NONE', #12681, 1000.000000000000000 ) ;
#14543=VECTOR ( 'NONE', #17071, 1000.000000000000000 ) ;
#14560=CARTESIAN_POINT ( 'NONE',  ( 1.136782529653004747, -40.00000000000000000, 3.000000000000000000 ) ) ;
#14567=DIRECTION ( 'NONE',  ( 0.000000000000000000, -0.000000000000000000, 1.000000000000000000 ) ) ;
#14577=EDGE_CURVE ( 'NONE', #13171, #1377, #11452, .T. ) ;
#14578=ORIENTED_EDGE ( 'NONE', *, *, #1816, .T. ) ;
#14611=DIRECTION ( 'NONE',  ( -1.000000000000000000, -0.000000000000000000, -0.000000000000000000 ) ) ;
#14613=CARTESIAN_POINT ( 'NONE',  ( 3.686287386450715076E-15, -16.60000000000000142, 25.01316734529526187 ) ) ;
#14617=VERTEX_POINT ( 'NONE', #16231 ) ;
#14649=VERTEX_POINT ( 'NONE', #10201 ) ;
#14663=FILL_AREA_STYLE_COLOUR ( '', #10566 ) ;
#14670=EDGE_CURVE ( 'NONE', #15279, #11185, #12714, .T. ) ;
#14693=ORIENTED_EDGE ( 'NONE', *, *, #14843, .T. ) ;
#14695=ORIENTED_EDGE ( 'NONE', *, *, #4413, .T. ) ;
#14699=PLANE ( 'NONE',  #3187 ) ;
#14720=ORIENTED_EDGE ( 'NONE', *, *, #14670, .T. ) ;
#14729=EDGE_CURVE ( 'NONE', #911, #18408, #11068, .T. ) ;
#14732=AXIS2_PLACEMENT_3D ( 'NONE', #46, #13328, #245 ) ;
#14744=AXIS2_PLACEMENT_3D ( 'NONE', #14560, #10069, #11693 ) ;
#14769=VERTEX_POINT ( 'NONE', #16797 ) ;
#14790=EDGE_LOOP ( 'NONE', ( #7451, #5731, #1517, #13071 ) ) ;
#14823=FACE_OUTER_BOUND ( 'NONE', #13730, .T. ) ;
#14825=( GEOMETRIC_REPRESENTATION_CONTEXT ( 3 ) GLOBAL_UNCERTAINTY_ASSIGNED_CONTEXT ( ( #3049 ) ) GLOBAL_UNIT_ASSIGNED_CONTEXT ( ( #15530, #8282, #2709 ) ) REPRESENTATION_CONTEXT ( 'NONE', 'WORKASPACE' ) );
#14843=EDGE_CURVE ( 'NONE', #13257, #11387, #11342, .T. ) ;
#14853=CARTESIAN_POINT ( 'NONE',  ( 15.00000000000000711, -45.00000000000000000, 6.000000000000000000 ) ) ;
#14865=VECTOR ( 'NONE', #10694, 1000.000000000000000 ) ;
#14881=DIRECTION ( 'NONE',  ( -0.000000000000000000, 1.000000000000000000, -0.000000000000000000 ) ) ;
#14910=EDGE_CURVE ( 'NONE', #998, #5396, #6171, .T. ) ;
#14943=DIRECTION ( 'NONE',  ( -0.000000000000000000, 1.000000000000000000, -0.000000000000000000 ) ) ;
#14956=CARTESIAN_POINT ( 'NONE',  ( -4.505465888036630062, -19.31487138727242581, 3.000000000000000000 ) ) ;
#14968=FACE_OUTER_BOUND ( 'NONE', #13168, .T. ) ;
#14988=PLANE ( 'NONE',  #13577 ) ;
#15007=VERTEX_POINT ( 'NONE', #2895 ) ;
#15038=VERTEX_POINT ( 'NONE', #4929 ) ;
#15043=SURFACE_STYLE_USAGE ( .BOTH. , #427 ) ;
#15080=ORIENTED_EDGE ( 'NONE', *, *, #16666, .T. ) ;
#15117=EDGE_CURVE ( 'NONE', #16909, #5705, #4840, .T. ) ;
#15127=DIRECTION ( 'NONE',  ( 0.8629742774544859607, -0.5052478564545405115, -0.000000000000000000 ) ) ;
#15170=AXIS2_PLACEMENT_3D ( 'NONE', #5871, #18343, #16908 ) ;
#15182=EDGE_CURVE ( 'NONE', #3563, #2803, #8449, .T. ) ;
#15187=ORIENTED_EDGE ( 'NONE', *, *, #11689, .T. ) ;
#15189=AXIS2_PLACEMENT_3D ( 'NONE', #8064, #789, #3364 ) ;
#15204=EDGE_CURVE ( 'NONE', #2316, #15038, #8357, .T. ) ;
#15218=CONICAL_SURFACE ( 'NONE', #16746, 2.100000000000000977, 1.029744258676656532 ) ;
#15236=( NAMED_UNIT ( * ) SI_UNIT ( $, .STERADIAN. ) SOLID_ANGLE_UNIT ( ) );
#15251=AXIS2_PLACEMENT_3D ( 'NONE', #3053, #11872, #2770 ) ;
#15256=MECHANICAL_DESIGN_GEOMETRIC_PRESENTATION_REPRESENTATION('',(#8236),#4882);
#15262=CARTESIAN_POINT ( 'NONE',  ( -4.999999999999995559, -30.00000000000000000, 31.00000000000000000 ) ) ;
#15272=ORIENTED_EDGE ( 'NONE', *, *, #11689, .F. ) ;
#15273=ORIENTED_EDGE ( 'NONE', *, *, #5347, .T. ) ;
#15279=VERTEX_POINT ( 'NONE', #12555 ) ;
#15281=EDGE_CURVE ( 'NONE', #15038, #14303, #11512, .T. ) ;
#15287=EDGE_CURVE ( 'NONE', #14370, #13171, #3258, .T. ) ;
#15290=CARTESIAN_POINT ( 'NONE',  ( 4.336808689942017736E-15, -27.00000000000000000, 31.00000000000000000 ) ) ;
#15350=CARTESIAN_POINT ( 'NONE',  ( 5.000000000000006217, -30.00000000000000000, 31.00000000000000000 ) ) ;
#15390=ORIENTED_EDGE ( 'NONE', *, *, #5077, .F. ) ;
#15392=DIRECTION ( 'NONE',  ( -0.000000000000000000, -0.000000000000000000, -1.000000000000000000 ) ) ;
#15399=LINE ( 'NONE', #5176, #12556 ) ;
#15471=CYLINDRICAL_SURFACE ( 'NONE', #15170, 2.100000000000000977 ) ;
#15497=AXIS2_PLACEMENT_3D ( 'NONE', #16772, #9130, #4736 ) ;
#15514=ADVANCED_FACE ( 'NONE', ( #3265 ), #9396, .T. ) ;
#15520=VERTEX_POINT ( 'NONE', #6627 ) ;
#15530=( LENGTH_UNIT ( ) NAMED_UNIT ( * ) SI_UNIT ( .MILLI., .METRE. ) );
#15566=CARTESIAN_POINT ( 'NONE',  ( -4.999999999999995559, -30.00000000000000000, 6.000000000000000000 ) ) ;
#15577=EDGE_CURVE ( 'NONE', #846, #5396, #8249, .T. ) ;
#15582=ORIENTED_EDGE ( 'NONE', *, *, #4041, .F. ) ;
#15595=CARTESIAN_POINT ( 'NONE',  ( -199.9999999999999716, -10.00000000000002665, 3.000000000000000000 ) ) ;
#15600=ADVANCED_FACE ( 'NONE', ( #17116, #1156, #8337 ), #18638, .F. ) ;
#15603=DIRECTION ( 'NONE',  ( -1.000000000000000000, -1.040834085586084257E-15, 0.000000000000000000 ) ) ;
#15606=DIRECTION ( 'NONE',  ( 0.000000000000000000, 0.000000000000000000, 1.000000000000000000 ) ) ;
#15608=ORIENTED_EDGE ( 'NONE', *, *, #14147, .T. ) ;
#15619=DIRECTION ( 'NONE',  ( -0.000000000000000000, -0.000000000000000000, 1.000000000000000000 ) ) ;
#15685=AXIS2_PLACEMENT_3D ( 'NONE', #12140, #6114, #10507 ) ;
#15686=LINE ( 'NONE', #14162, #7624 ) ;
#15687=CARTESIAN_POINT ( 'NONE',  ( 5.000000000000004441, -27.00000000000000000, 26.00000000000000000 ) ) ;
#15716=CARTESIAN_POINT ( 'NONE',  ( 0.000000000000000000, 0.000000000000000000, 0.000000000000000000 ) ) ;
#15726=VERTEX_POINT ( 'NONE', #11669 ) ;
#15733=ORIENTED_EDGE ( 'NONE', *, *, #11083, .F. ) ;
#15736=LINE ( 'NONE', #14219, #9277 ) ;
#15744=AXIS2_PLACEMENT_3D ( 'NONE', #17657, #4561, #12113 ) ;
#15774=CIRCLE ( 'NONE', #9381, 5.000000000000000888 ) ;
#15782=VERTEX_POINT ( 'NONE', #10038 ) ;
#15840=EDGE_CURVE ( 'NONE', #15520, #3962, #4789, .T. ) ;
#15842=DIRECTION ( 'NONE',  ( -1.000000000000000000, -0.000000000000000000, -0.000000000000000000 ) ) ;
#15857=DIRECTION ( 'NONE',  ( -1.000000000000000000, 0.000000000000000000, 0.000000000000000000 ) ) ;
#15888=ORIENTED_EDGE ( 'NONE', *, *, #13925, .F. ) ;
#15908=DIRECTION ( 'NONE',  ( -0.000000000000000000, 1.000000000000000000, -0.000000000000000000 ) ) ;
#15938=ORIENTED_EDGE ( 'NONE', *, *, #17349, .T. ) ;
#15948=CYLINDRICAL_SURFACE ( 'NONE', #4408, 5.000000000000000000 ) ;
#15970=CYLINDRICAL_SURFACE ( 'NONE', #15251, 5.000000000000000888 ) ;
#16037=ORIENTED_EDGE ( 'NONE', *, *, #9265, .F. ) ;
#16051=DIRECTION ( 'NONE',  ( 0.000000000000000000, 0.5150380749100523792, 0.8571673007021134438 ) ) ;
#16125=CARTESIAN_POINT ( 'NONE',  ( -27.50000000000000711, -12.50000000000000178, 6.000000000000000000 ) ) ;
#16134=ORIENTED_EDGE ( 'NONE', *, *, #2270, .F. ) ;
#16146=PLANE ( 'NONE',  #167 ) ;
#16196=DIRECTION ( 'NONE',  ( -0.000000000000000000, 0.000000000000000000, 1.000000000000000000 ) ) ;
#16231=CARTESIAN_POINT ( 'NONE',  ( -4.999999999999995559, -30.00000000000000000, 6.000000000000000000 ) ) ;
#16247=CARTESIAN_POINT ( 'NONE',  ( -0.2192422490275049152, -45.00000000000000000, 3.000000000000000000 ) ) ;
#16274=ORIENTED_EDGE ( 'NONE', *, *, #15840, .T. ) ;
#16294=VECTOR ( 'NONE', #15127, 1000.000000000000227 ) ;
#16438=CARTESIAN_POINT ( 'NONE',  ( -30.00000000000000355, -12.50000000000000178, 6.000000000000000000 ) ) ;
#16441=CARTESIAN_POINT ( 'NONE',  ( 20.00000000000000711, -40.00000000000000000, 6.000000000000000000 ) ) ;
#16465=ORIENTED_EDGE ( 'NONE', *, *, #5347, .F. ) ;
#16471=VECTOR ( 'NONE', #4706, 1000.000000000000227 ) ;
#16475=CARTESIAN_POINT ( 'NONE',  ( -3.335251384444446021, -19.99999999999999645, 3.000000000000000000 ) ) ;
#16481=COLOUR_RGB ( '', 0.09019608, 0.27058824, 0.51372549) ;
#16530=ORIENTED_EDGE ( 'NONE', *, *, #3603, .F. ) ;
#16556=DIRECTION ( 'NONE',  ( 0.5052478564545405115, 0.8629742774544859607, -0.000000000000000000 ) ) ;
#16619=CIRCLE ( 'NONE', #7469, 2.499999999999995115 ) ;
#16622=DIRECTION ( 'NONE',  ( 1.000000000000000000, 0.000000000000000000, 0.000000000000000000 ) ) ;
#16640=VECTOR ( 'NONE', #10611, 1000.000000000000000 ) ;
#16643=ORIENTED_EDGE ( 'NONE', *, *, #3271, .T. ) ;
#16665=FACE_OUTER_BOUND ( 'NONE', #10901, .T. ) ;
#16666=EDGE_CURVE ( 'NONE', #4207, #5898, #9680, .T. ) ;
#16716=DIRECTION ( 'NONE',  ( 1.000000000000000000, 0.000000000000000000, 0.000000000000000000 ) ) ;
#16746=AXIS2_PLACEMENT_3D ( 'NONE', #4627, #14943, #3565 ) ;
#16756=ORIENTED_EDGE ( 'NONE', *, *, #12638, .F. ) ;
#16757=DIRECTION ( 'NONE',  ( -0.000000000000000000, -0.000000000000000000, 1.000000000000000000 ) ) ;
#16772=CARTESIAN_POINT ( 'NONE',  ( -55.93192566395838128, 4.999999999999974243, 6.000000000000000000 ) ) ;
#16780=ORIENTED_EDGE ( 'NONE', *, *, #18168, .T. ) ;
#16781=EDGE_CURVE ( 'NONE', #3169, #998, #11227, .T. ) ;
#16797=CARTESIAN_POINT ( 'NONE',  ( 3.686287386450715076E-15, -27.00000000000000000, 21.01316734529526187 ) ) ;
#16809=EDGE_CURVE ( 'NONE', #9356, #11185, #15686, .T. ) ;
#16814=EDGE_CURVE ( 'NONE', #2805, #14769, #9850, .T. ) ;
#16851=DIRECTION ( 'NONE',  ( -0.000000000000000000, -1.000000000000000000, -0.000000000000000000 ) ) ;
#16853=DIRECTION ( 'NONE',  ( -0.000000000000000000, -1.000000000000000000, -0.000000000000000000 ) ) ;
#16868=ORIENTED_EDGE ( 'NONE', *, *, #4644, .F. ) ;
#16898=AXIS2_PLACEMENT_3D ( 'NONE', #11856, #2, #6028 ) ;
#16907=ORIENTED_EDGE ( 'NONE', *, *, #4135, .F. ) ;
#16908=DIRECTION ( 'NONE',  ( 0.000000000000000000, 0.000000000000000000, 1.000000000000000000 ) ) ;
#16909=VERTEX_POINT ( 'NONE', #17219 ) ;
#16926=DIRECTION ( 'NONE',  ( 0.000000000000000000, -1.000000000000000000, 0.000000000000000000 ) ) ;
#16933=ORIENTED_EDGE ( 'NONE', *, *, #17349, .F. ) ;
#16944=VECTOR ( 'NONE', #16926, 1000.000000000000000 ) ;
#16960=FACE_OUTER_BOUND ( 'NONE', #8186, .T. ) ;
#16962=EDGE_LOOP ( 'NONE', ( #7919, #6725, #8615, #4648 ) ) ;
#16971=DIRECTION ( 'NONE',  ( 0.000000000000000000, 0.000000000000000000, -1.000000000000000000 ) ) ;
#16987=AXIS2_PLACEMENT_3D ( 'NONE', #11956, #5822, #12053 ) ;
#16996=VECTOR ( 'NONE', #6323, 1000.000000000000000 ) ;
#17014=EDGE_CURVE ( 'NONE', #9580, #15726, #6337, .T. ) ;
#17034=AXIS2_PLACEMENT_3D ( 'NONE', #17225, #18383, #15603 ) ;
#17052=DIRECTION ( 'NONE',  ( 0.000000000000000000, 0.000000000000000000, 1.000000000000000000 ) ) ;
#17071=DIRECTION ( 'NONE',  ( -1.000000000000000000, -0.000000000000000000, -0.000000000000000000 ) ) ;
#17096=ORIENTED_EDGE ( 'NONE', *, *, #4769, .T. ) ;
#17116=FACE_BOUND ( 'NONE', #5870, .T. ) ;
#17147=EDGE_LOOP ( 'NONE', ( #17802, #7887 ) ) ;
#17164=DIRECTION ( 'NONE',  ( 0.000000000000000000, -1.000000000000000000, 0.000000000000000000 ) ) ;
#17166=DIRECTION ( 'NONE',  ( -1.000000000000000000, 0.000000000000000000, 0.000000000000000000 ) ) ;
#17176=DIRECTION ( 'NONE',  ( 0.000000000000000000, 0.000000000000000000, -1.000000000000000000 ) ) ;
#17201=DIRECTION ( 'NONE',  ( -0.000000000000000000, 1.000000000000000000, -0.000000000000000000 ) ) ;
#17206=DIRECTION ( 'NONE',  ( 0.000000000000000000, 0.000000000000000000, -1.000000000000000000 ) ) ;
#17219=CARTESIAN_POINT ( 'NONE',  ( -61.35602477868047799, -10.00000000000000888, 3.000000000000000000 ) ) ;
#17225=CARTESIAN_POINT ( 'NONE',  ( -1.979226605763932723, -14.99999999999999645, 3.000000000000000000 ) ) ;
#17226=DIRECTION ( 'NONE',  ( -0.000000000000000000, -0.000000000000000000, -1.000000000000000000 ) ) ;
#17227=DIRECTION ( 'NONE',  ( 0.000000000000000000, 0.000000000000000000, 1.000000000000000000 ) ) ;
#17228=DIRECTION ( 'NONE',  ( 1.000000000000000000, 0.000000000000000000, 0.000000000000000000 ) ) ;
#17248=AXIS2_PLACEMENT_3D ( 'NONE', #3310, #1897, #4570 ) ;
#17249=DIRECTION ( 'NONE',  ( 1.000000000000000000, 0.000000000000000000, 0.000000000000000000 ) ) ;
#17253=ORIENTED_EDGE ( 'NONE', *, *, #6802, .F. ) ;
#17268=CARTESIAN_POINT ( 'NONE',  ( 0.000000000000000000, 0.000000000000000000, 3.000000000000000000 ) ) ;
#17273=EDGE_CURVE ( 'NONE', #14769, #2548, #3675, .T. ) ;
#17283=CARTESIAN_POINT ( 'NONE',  ( -199.9999999999999716, 4.999999999999973355, 6.000000000000000000 ) ) ;
#17284=CARTESIAN_POINT ( 'NONE',  ( 20.00000000000000711, -19.99999999999999645, 6.000000000000000000 ) ) ;
#17323=DIRECTION ( 'NONE',  ( -1.000000000000000000, 0.000000000000000000, 0.000000000000000000 ) ) ;
#17339=CARTESIAN_POINT ( 'NONE',  ( -194.9999999999999716, 4.999999999999973355, 6.000000000000000000 ) ) ;
#17344=CARTESIAN_POINT ( 'NONE',  ( 4.336808689942017736E-15, 0.000000000000000000, 26.00000000000000000 ) ) ;
#17348=ADVANCED_FACE ( 'NONE', ( #5911 ), #1717, .F. ) ;
#17349=EDGE_CURVE ( 'NONE', #6600, #182, #484, .T. ) ;
#17360=EDGE_CURVE ( 'NONE', #5898, #4207, #5463, .T. ) ;
#17371=VECTOR ( 'NONE', #4758, 1000.000000000000000 ) ;
#17382=DIRECTION ( 'NONE',  ( 0.000000000000000000, 0.000000000000000000, -1.000000000000000000 ) ) ;
#17385=CARTESIAN_POINT ( 'NONE',  ( -199.9999999999999716, 9.999999999999973355, 6.000000000000000000 ) ) ;
#17411=CARTESIAN_POINT ( 'NONE',  ( -4.999999999999995559, -30.00000000000000000, 31.00000000000000000 ) ) ;
#17434=ORIENTED_EDGE ( 'NONE', *, *, #8575, .F. ) ;
#17474=EDGE_CURVE ( 'NONE', #15726, #5898, #11633, .T. ) ;
#17506=CARTESIAN_POINT ( 'NONE',  ( 3.686287386450715076E-15, -16.60000000000000142, 21.01316734529526187 ) ) ;
#17508=AXIS2_PLACEMENT_3D ( 'NONE', #2689, #17226, #17323 ) ;
#17536=( NAMED_UNIT ( * ) SI_UNIT ( $, .STERADIAN. ) SOLID_ANGLE_UNIT ( ) );
#17538=DIRECTION ( 'NONE',  ( 0.000000000000000000, -0.000000000000000000, -1.000000000000000000 ) ) ;
#17546=CARTESIAN_POINT ( 'NONE',  ( -61.35602477868047799, -10.00000000000000888, 6.000000000000000000 ) ) ;
#17610=AXIS2_PLACEMENT_3D ( 'NONE', #836, #10886, #2356 ) ;
#17657=CARTESIAN_POINT ( 'NONE',  ( 5.000000000000006217, -30.00000000000000000, 31.00000000000000000 ) ) ;
#17677=ORIENTED_EDGE ( 'NONE', *, *, #15182, .F. ) ;
#17699=VECTOR ( 'NONE', #1454, 1000.000000000000000 ) ;
#17735=DIRECTION ( 'NONE',  ( 1.000000000000000000, 1.239088197126290570E-16, -0.000000000000000000 ) ) ;
#17739=DIRECTION ( 'NONE',  ( 0.000000000000000000, -1.000000000000000000, 0.000000000000000000 ) ) ;
#17768=ORIENTED_EDGE ( 'NONE', *, *, #8646, .T. ) ;
#17802=ORIENTED_EDGE ( 'NONE', *, *, #4644, .T. ) ;
#17824=VECTOR ( 'NONE', #6619, 1000.000000000000000 ) ;
#17863=ORIENTED_EDGE ( 'NONE', *, *, #375, .T. ) ;
#17868=VECTOR ( 'NONE', #13325, 1000.000000000000000 ) ;
#17877=EDGE_CURVE ( 'NONE', #14649, #16909, #3179, .T. ) ;
#17881=EDGE_CURVE ( 'NONE', #10186, #12673, #7321, .T. ) ;
#17901=ADVANCED_FACE ( 'NONE', ( #14469 ), #5863, .F. ) ;
#17924=DIRECTION ( 'NONE',  ( 0.000000000000000000, -1.000000000000000000, 0.000000000000000000 ) ) ;
#17937=AXIS2_PLACEMENT_3D ( 'NONE', #2335, #15606, #17228 ) ;
#17956=LINE ( 'NONE', #171, #17371 ) ;
#17966=ORIENTED_EDGE ( 'NONE', *, *, #4413, .F. ) ;
#17972=CARTESIAN_POINT ( 'NONE',  ( -1.979226605763932723, -14.99999999999999645, 6.000000000000000000 ) ) ;
#18014=VERTEX_POINT ( 'NONE', #5360 ) ;
#18036=LINE ( 'NONE', #10773, #6608 ) ;
#18060=ORIENTED_EDGE ( 'NONE', *, *, #15117, .F. ) ;
#18088=EDGE_CURVE ( 'NONE', #5678, #3563, #10664, .T. ) ;
#18114=ADVANCED_BREP_SHAPE_REPRESENTATION ( '', ( #3553, #2030 ), #14825 ) ;
#18129=EDGE_CURVE ( 'NONE', #2803, #15520, #14337, .T. ) ;
#18168=EDGE_CURVE ( 'NONE', #9580, #12603, #1150, .T. ) ;
#18185=ORIENTED_EDGE ( 'NONE', *, *, #2382, .T. ) ;
#18216=CIRCLE ( 'NONE', #11817, 4.999999999999997335 ) ;
#18254=CARTESIAN_POINT ( 'NONE',  ( -32.49999999999999289, -12.50000000000000178, 3.000000000000000000 ) ) ;
#18266=FACE_OUTER_BOUND ( 'NONE', #5541, .T. ) ;
#18276=ORIENTED_EDGE ( 'NONE', *, *, #1816, .F. ) ;
#18334=CARTESIAN_POINT ( 'NONE',  ( -1.389456752619696367, -44.31487138727242581, 6.000000000000000000 ) ) ;
#18341=ORIENTED_EDGE ( 'NONE', *, *, #13748, .T. ) ;
#18343=DIRECTION ( 'NONE',  ( -0.000000000000000000, 1.000000000000000000, -0.000000000000000000 ) ) ;
#18383=DIRECTION ( 'NONE',  ( -0.000000000000000000, -0.000000000000000000, 1.000000000000000000 ) ) ;
#18385=DIRECTION ( 'NONE',  ( -0.000000000000000000, -0.000000000000000000, 1.000000000000000000 ) ) ;
#18395=LINE ( 'NONE', #11147, #5319 ) ;
#18408=VERTEX_POINT ( 'NONE', #18334 ) ;
#18451=ORIENTED_EDGE ( 'NONE', *, *, #16814, .T. ) ;
#18480=DIRECTION ( 'NONE',  ( -1.000000000000000000, -1.239088197126290570E-16, 0.000000000000000000 ) ) ;
#18485=ORIENTED_EDGE ( 'NONE', *, *, #14670, .F. ) ;
#18489=AXIS2_PLACEMENT_3D ( 'NONE', #3048, #16556, #1735 ) ;
#18528=ORIENTED_EDGE ( 'NONE', *, *, #14729, .F. ) ;
#18555=DIRECTION ( 'NONE',  ( -1.000000000000000000, 0.000000000000000000, 0.000000000000000000 ) ) ;
#18607=DIRECTION ( 'NONE',  ( -1.000000000000000000, 0.000000000000000000, -0.000000000000000000 ) ) ;
#18638=PLANE ( 'NONE',  #9391 ) ;
#18720=CARTESIAN_POINT ( 'NONE',  ( -4.999999999999995559, -30.00000000000000000, 26.00000000000000000 ) ) ;
#18741=ADVANCED_FACE ( 'NONE', ( #7641 ), #5890, .T. ) ;
#18753=VECTOR ( 'NONE', #8856, 1000.000000000000000 ) ;
#18767=ORIENTED_EDGE ( 'NONE', *, *, #16809, .F. ) ;
#18770=CIRCLE ( 'NONE', #10859, 5.000000000000000888 ) ;
#18811=CARTESIAN_POINT ( 'NONE',  ( -3.335251384444446021, -19.99999999999999645, 6.000000000000000000 ) ) ;
#18812=DIRECTION ( 'NONE',  ( -0.8629742774544855166, 0.5052478564545411777, -0.000000000000000000 ) ) ;
#18818=LINE ( 'NONE', #16247, #738 ) ;
#18824=AXIS2_PLACEMENT_3D ( 'NONE', #8084, #3959, #17052 ) ;
#18836=ADVANCED_FACE ( 'NONE', ( #3782 ), #10972, .T. ) ;
#18846=VERTEX_POINT ( 'NONE', #10882 ) ;
#18875=ORIENTED_EDGE ( 'NONE', *, *, #18168, .F. ) ;
#18878=ORIENTED_EDGE ( 'NONE', *, *, #5489, .F. ) ;
#18886=ADVANCED_FACE ( 'NONE', ( #13913 ), #3604, .F. ) ;
ENDSEC;
END-ISO-10303-21;
